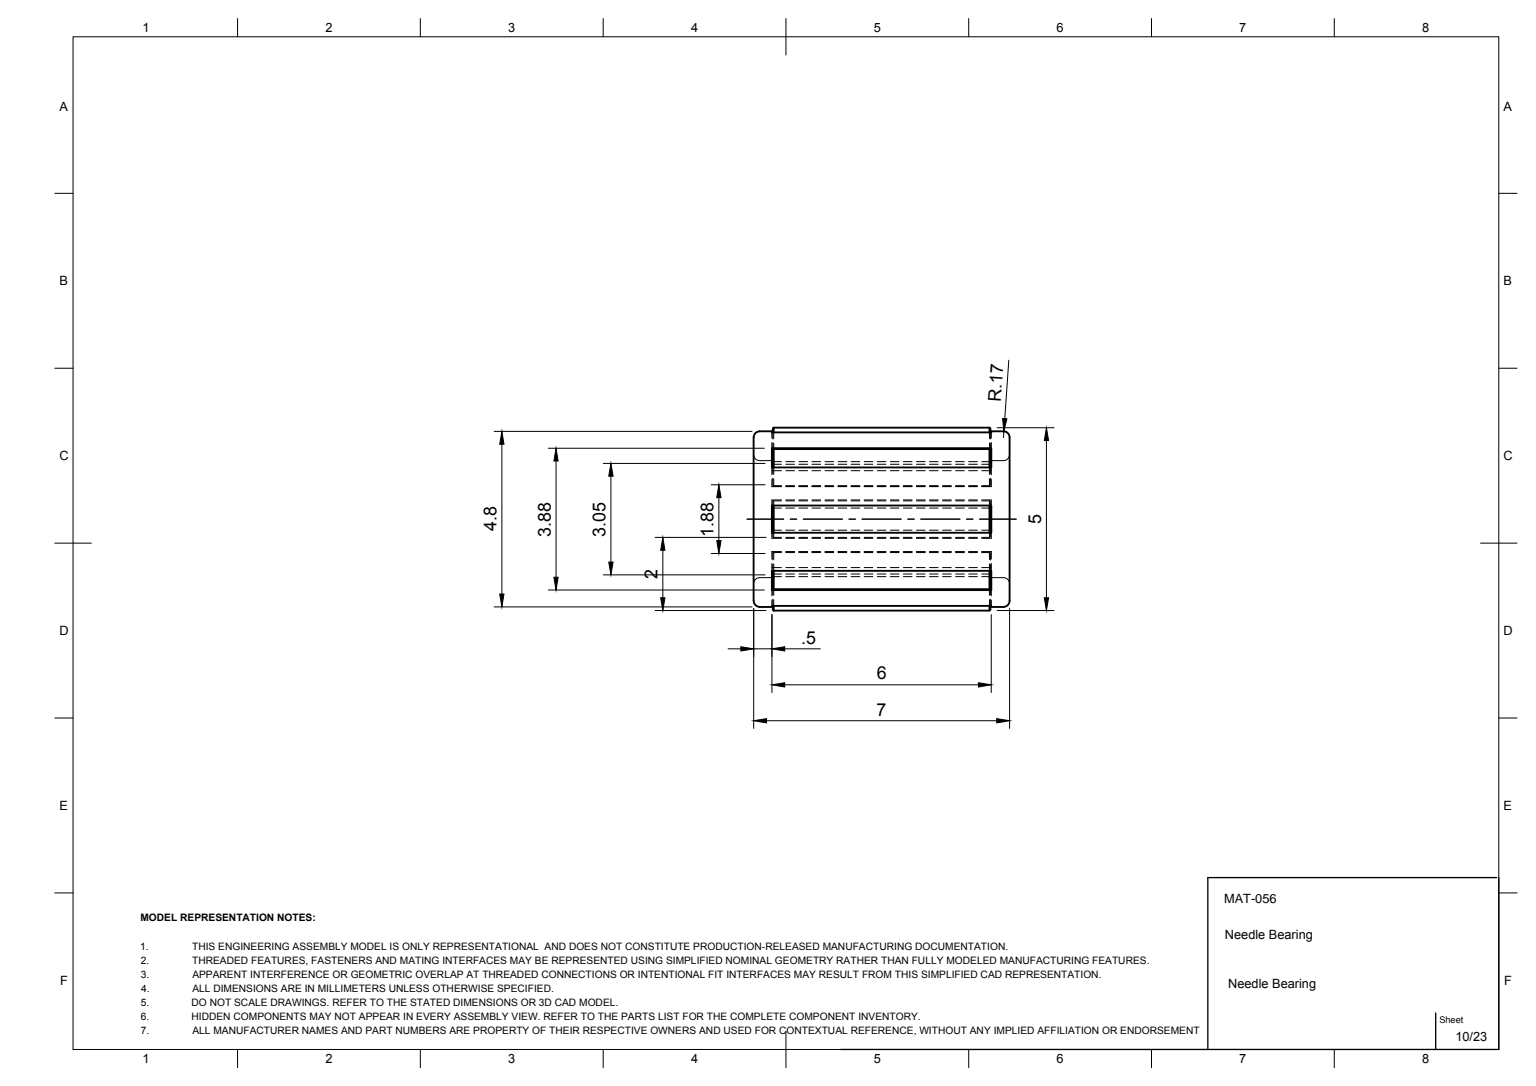
ISO-10303-21;
HEADER;
/* Generated by software containing ST-Developer
 * from STEP Tools, Inc. (www.steptools.com) 
 */

FILE_DESCRIPTION(
/* description */ (''),
/* implementation_level */ '2;1');

FILE_NAME(
/* name */ 'Needle Bearing.step',
/* time_stamp */ '2026-10-28T16:47:13+01:00',
/* author */ (''),
/* organization */ (''),
/* preprocessor_version */ 'ST-DEVELOPER v20.2',
/* originating_system */ 'Autodesk Translation Framework v15.17.0.0',
/* authorisation */ '');

FILE_SCHEMA (('AUTOMOTIVE_DESIGN { 1 0 10303 214 3 1 1 }'));
ENDSEC;

DATA;
#10=MECHANICAL_DESIGN_GEOMETRIC_PRESENTATION_REPRESENTATION('',(#4578,#4579,#4580,#4581,#4582,#4583,#4584,#4585,#4586),#459242);
#1858=TOROIDAL_SURFACE('',#98857,1.76666666666667,0.166666666666667);
#1859=TOROIDAL_SURFACE('',#98884,2.23333333333333,0.166666666666667);
#1860=TOROIDAL_SURFACE('',#98908,2.23333333333333,0.166666666666667);
#1861=TOROIDAL_SURFACE('',#98913,1.76666666666667,0.166666666666667);
#4413=SHAPE_REPRESENTATION_RELATIONSHIP('SRR','None',#459338,#4434);
#4434=ADVANCED_BREP_SHAPE_REPRESENTATION('',(#4458,#4459,#4460,#4461,#4462,
#4463,#4464,#4465,#4466),#459227);
#4458=MANIFOLD_SOLID_BREP('Bearing body',#94636);
#4459=MANIFOLD_SOLID_BREP('Roller 1',#94637);
#4460=MANIFOLD_SOLID_BREP('Roller 2',#94638);
#4461=MANIFOLD_SOLID_BREP('Roller 3',#94639);
#4462=MANIFOLD_SOLID_BREP('Roller 4',#94640);
#4463=MANIFOLD_SOLID_BREP('Roller 5',#94641);
#4464=MANIFOLD_SOLID_BREP('Roller 6',#94642);
#4465=MANIFOLD_SOLID_BREP('Roller 7',#94643);
#4466=MANIFOLD_SOLID_BREP('Roller 8',#94644);
#4578=STYLED_ITEM('',(#459526),#4458);
#4579=STYLED_ITEM('',(#459526),#4459);
#4580=STYLED_ITEM('',(#459526),#4460);
#4581=STYLED_ITEM('',(#459526),#4461);
#4582=STYLED_ITEM('',(#459526),#4462);
#4583=STYLED_ITEM('',(#459526),#4463);
#4584=STYLED_ITEM('',(#459526),#4464);
#4585=STYLED_ITEM('',(#459526),#4465);
#4586=STYLED_ITEM('',(#459526),#4466);
#4861=CONICAL_SURFACE('',#98979,0.4875,0.785398163397448);
#4862=CONICAL_SURFACE('',#98985,0.4875,0.785398163397448);
#4863=CONICAL_SURFACE('',#98988,0.4875,0.785398163397492);
#4864=CONICAL_SURFACE('',#98994,0.4875,0.785398163397492);
#4865=CONICAL_SURFACE('',#98997,0.4875,0.785398163397448);
#4866=CONICAL_SURFACE('',#99003,0.4875,0.785398163397448);
#4867=CONICAL_SURFACE('',#99006,0.4875,0.78539816339745);
#4868=CONICAL_SURFACE('',#99012,0.4875,0.78539816339745);
#4869=CONICAL_SURFACE('',#99015,0.4875,0.785398163397448);
#4870=CONICAL_SURFACE('',#99021,0.4875,0.785398163397448);
#4871=CONICAL_SURFACE('',#99024,0.4875,0.78539816339745);
#4872=CONICAL_SURFACE('',#99030,0.4875,0.78539816339745);
#4873=CONICAL_SURFACE('',#99033,0.4875,0.785398163397448);
#4874=CONICAL_SURFACE('',#99039,0.4875,0.785398163397448);
#4875=CONICAL_SURFACE('',#99042,0.4875,0.78539816339745);
#4876=CONICAL_SURFACE('',#99048,0.4875,0.78539816339745);
#5193=FACE_BOUND('',#14123,.T.);
#5194=FACE_BOUND('',#14125,.T.);
#5195=FACE_BOUND('',#14126,.T.);
#5196=FACE_BOUND('',#14127,.T.);
#5197=FACE_BOUND('',#14128,.T.);
#5198=FACE_BOUND('',#14129,.T.);
#5199=FACE_BOUND('',#14130,.T.);
#5200=FACE_BOUND('',#14131,.T.);
#5201=FACE_BOUND('',#14134,.T.);
#5202=FACE_BOUND('',#14135,.T.);
#5203=FACE_BOUND('',#14136,.T.);
#5204=FACE_BOUND('',#14137,.T.);
#5205=FACE_BOUND('',#14138,.T.);
#5206=FACE_BOUND('',#14139,.T.);
#5207=FACE_BOUND('',#14140,.T.);
#5208=FACE_BOUND('',#14143,.T.);
#5650=PLANE('',#98861);
#5651=PLANE('',#98911);
#5652=PLANE('',#98915);
#5653=PLANE('',#98920);
#5654=PLANE('',#98923);
#5655=PLANE('',#98928);
#5656=PLANE('',#98931);
#5657=PLANE('',#98936);
#5658=PLANE('',#98939);
#5659=PLANE('',#98944);
#5660=PLANE('',#98947);
#5661=PLANE('',#98952);
#5662=PLANE('',#98955);
#5663=PLANE('',#98960);
#5664=PLANE('',#98963);
#5665=PLANE('',#98968);
#5666=PLANE('',#98971);
#5667=PLANE('',#98976);
#5668=PLANE('',#98984);
#5669=PLANE('',#98987);
#5670=PLANE('',#98993);
#5671=PLANE('',#98996);
#5672=PLANE('',#99002);
#5673=PLANE('',#99005);
#5674=PLANE('',#99011);
#5675=PLANE('',#99014);
#5676=PLANE('',#99020);
#5677=PLANE('',#99023);
#5678=PLANE('',#99029);
#5679=PLANE('',#99032);
#5680=PLANE('',#99038);
#5681=PLANE('',#99041);
#5682=PLANE('',#99047);
#5683=PLANE('',#99050);
#8233=FACE_OUTER_BOUND('',#14121,.T.);
#8234=FACE_OUTER_BOUND('',#14122,.T.);
#8235=FACE_OUTER_BOUND('',#14124,.T.);
#8236=FACE_OUTER_BOUND('',#14132,.T.);
#8237=FACE_OUTER_BOUND('',#14133,.T.);
#8238=FACE_OUTER_BOUND('',#14141,.T.);
#8239=FACE_OUTER_BOUND('',#14142,.T.);
#8240=FACE_OUTER_BOUND('',#14144,.T.);
#8241=FACE_OUTER_BOUND('',#14145,.T.);
#8242=FACE_OUTER_BOUND('',#14146,.T.);
#8243=FACE_OUTER_BOUND('',#14147,.T.);
#8244=FACE_OUTER_BOUND('',#14148,.T.);
#8245=FACE_OUTER_BOUND('',#14149,.T.);
#8246=FACE_OUTER_BOUND('',#14150,.T.);
#8247=FACE_OUTER_BOUND('',#14151,.T.);
#8248=FACE_OUTER_BOUND('',#14152,.T.);
#8249=FACE_OUTER_BOUND('',#14153,.T.);
#8250=FACE_OUTER_BOUND('',#14154,.T.);
#8251=FACE_OUTER_BOUND('',#14155,.T.);
#8252=FACE_OUTER_BOUND('',#14156,.T.);
#8253=FACE_OUTER_BOUND('',#14157,.T.);
#8254=FACE_OUTER_BOUND('',#14158,.T.);
#8255=FACE_OUTER_BOUND('',#14159,.T.);
#8256=FACE_OUTER_BOUND('',#14160,.T.);
#8257=FACE_OUTER_BOUND('',#14161,.T.);
#8258=FACE_OUTER_BOUND('',#14162,.T.);
#8259=FACE_OUTER_BOUND('',#14163,.T.);
#8260=FACE_OUTER_BOUND('',#14164,.T.);
#8261=FACE_OUTER_BOUND('',#14165,.T.);
#8262=FACE_OUTER_BOUND('',#14166,.T.);
#8263=FACE_OUTER_BOUND('',#14167,.T.);
#8264=FACE_OUTER_BOUND('',#14168,.T.);
#8265=FACE_OUTER_BOUND('',#14169,.T.);
#8266=FACE_OUTER_BOUND('',#14170,.T.);
#8267=FACE_OUTER_BOUND('',#14171,.T.);
#8268=FACE_OUTER_BOUND('',#14172,.T.);
#8269=FACE_OUTER_BOUND('',#14173,.T.);
#8270=FACE_OUTER_BOUND('',#14174,.T.);
#8271=FACE_OUTER_BOUND('',#14175,.T.);
#8272=FACE_OUTER_BOUND('',#14176,.T.);
#8273=FACE_OUTER_BOUND('',#14177,.T.);
#8274=FACE_OUTER_BOUND('',#14178,.T.);
#8275=FACE_OUTER_BOUND('',#14179,.T.);
#8276=FACE_OUTER_BOUND('',#14180,.T.);
#8277=FACE_OUTER_BOUND('',#14181,.T.);
#8278=FACE_OUTER_BOUND('',#14182,.T.);
#8279=FACE_OUTER_BOUND('',#14183,.T.);
#8280=FACE_OUTER_BOUND('',#14184,.T.);
#8281=FACE_OUTER_BOUND('',#14185,.T.);
#8282=FACE_OUTER_BOUND('',#14186,.T.);
#8283=FACE_OUTER_BOUND('',#14187,.T.);
#8284=FACE_OUTER_BOUND('',#14188,.T.);
#8285=FACE_OUTER_BOUND('',#14189,.T.);
#8286=FACE_OUTER_BOUND('',#14190,.T.);
#8287=FACE_OUTER_BOUND('',#14191,.T.);
#8288=FACE_OUTER_BOUND('',#14192,.T.);
#8289=FACE_OUTER_BOUND('',#14193,.T.);
#8290=FACE_OUTER_BOUND('',#14194,.T.);
#8291=FACE_OUTER_BOUND('',#14195,.T.);
#8292=FACE_OUTER_BOUND('',#14196,.T.);
#8293=FACE_OUTER_BOUND('',#14197,.T.);
#8294=FACE_OUTER_BOUND('',#14198,.T.);
#8295=FACE_OUTER_BOUND('',#14199,.T.);
#8296=FACE_OUTER_BOUND('',#14200,.T.);
#8297=FACE_OUTER_BOUND('',#14201,.T.);
#8298=FACE_OUTER_BOUND('',#14202,.T.);
#8299=FACE_OUTER_BOUND('',#14203,.T.);
#8300=FACE_OUTER_BOUND('',#14204,.T.);
#8301=FACE_OUTER_BOUND('',#14205,.T.);
#8302=FACE_OUTER_BOUND('',#14206,.T.);
#8303=FACE_OUTER_BOUND('',#14207,.T.);
#8304=FACE_OUTER_BOUND('',#14208,.T.);
#8305=FACE_OUTER_BOUND('',#14209,.T.);
#8306=FACE_OUTER_BOUND('',#14210,.T.);
#8307=FACE_OUTER_BOUND('',#14211,.T.);
#8308=FACE_OUTER_BOUND('',#14212,.T.);
#8309=FACE_OUTER_BOUND('',#14213,.T.);
#8310=FACE_OUTER_BOUND('',#14214,.T.);
#8311=FACE_OUTER_BOUND('',#14215,.T.);
#8312=FACE_OUTER_BOUND('',#14216,.T.);
#14121=EDGE_LOOP('',(#68422,#68423,#68424,#68425));
#14122=EDGE_LOOP('',(#68426));
#14123=EDGE_LOOP('',(#68427));
#14124=EDGE_LOOP('',(#68428,#68429,#68430,#68431,#68432,#68433,#68434,#68435,
#68436,#68437,#68438,#68439,#68440));
#14125=EDGE_LOOP('',(#68441,#68442,#68443,#68444));
#14126=EDGE_LOOP('',(#68445,#68446,#68447,#68448));
#14127=EDGE_LOOP('',(#68449,#68450,#68451,#68452));
#14128=EDGE_LOOP('',(#68453,#68454,#68455,#68456));
#14129=EDGE_LOOP('',(#68457,#68458,#68459,#68460));
#14130=EDGE_LOOP('',(#68461,#68462,#68463,#68464));
#14131=EDGE_LOOP('',(#68465,#68466,#68467,#68468));
#14132=EDGE_LOOP('',(#68469,#68470,#68471,#68472,#68473));
#14133=EDGE_LOOP('',(#68474,#68475,#68476,#68477,#68478,#68479,#68480,#68481,
#68482,#68483,#68484,#68485,#68486));
#14134=EDGE_LOOP('',(#68487,#68488,#68489,#68490));
#14135=EDGE_LOOP('',(#68491,#68492,#68493,#68494));
#14136=EDGE_LOOP('',(#68495,#68496,#68497,#68498));
#14137=EDGE_LOOP('',(#68499,#68500,#68501,#68502));
#14138=EDGE_LOOP('',(#68503,#68504,#68505,#68506));
#14139=EDGE_LOOP('',(#68507,#68508,#68509,#68510));
#14140=EDGE_LOOP('',(#68511,#68512,#68513,#68514));
#14141=EDGE_LOOP('',(#68515,#68516,#68517,#68518));
#14142=EDGE_LOOP('',(#68519));
#14143=EDGE_LOOP('',(#68520));
#14144=EDGE_LOOP('',(#68521,#68522,#68523,#68524,#68525));
#14145=EDGE_LOOP('',(#68526,#68527,#68528,#68529));
#14146=EDGE_LOOP('',(#68530,#68531,#68532,#68533));
#14147=EDGE_LOOP('',(#68534,#68535,#68536,#68537));
#14148=EDGE_LOOP('',(#68538,#68539,#68540,#68541));
#14149=EDGE_LOOP('',(#68542,#68543,#68544,#68545));
#14150=EDGE_LOOP('',(#68546,#68547,#68548,#68549));
#14151=EDGE_LOOP('',(#68550,#68551,#68552,#68553));
#14152=EDGE_LOOP('',(#68554,#68555,#68556,#68557));
#14153=EDGE_LOOP('',(#68558,#68559,#68560,#68561));
#14154=EDGE_LOOP('',(#68562,#68563,#68564,#68565));
#14155=EDGE_LOOP('',(#68566,#68567,#68568,#68569));
#14156=EDGE_LOOP('',(#68570,#68571,#68572,#68573));
#14157=EDGE_LOOP('',(#68574,#68575,#68576,#68577,#68578,#68579));
#14158=EDGE_LOOP('',(#68580,#68581,#68582,#68583));
#14159=EDGE_LOOP('',(#68584,#68585,#68586,#68587,#68588,#68589));
#14160=EDGE_LOOP('',(#68590,#68591,#68592,#68593));
#14161=EDGE_LOOP('',(#68594,#68595,#68596,#68597));
#14162=EDGE_LOOP('',(#68598,#68599,#68600,#68601));
#14163=EDGE_LOOP('',(#68602,#68603,#68604,#68605));
#14164=EDGE_LOOP('',(#68606,#68607,#68608,#68609));
#14165=EDGE_LOOP('',(#68610,#68611,#68612,#68613));
#14166=EDGE_LOOP('',(#68614,#68615,#68616,#68617));
#14167=EDGE_LOOP('',(#68618,#68619,#68620,#68621));
#14168=EDGE_LOOP('',(#68622,#68623,#68624,#68625));
#14169=EDGE_LOOP('',(#68626,#68627,#68628,#68629));
#14170=EDGE_LOOP('',(#68630,#68631,#68632,#68633));
#14171=EDGE_LOOP('',(#68634,#68635,#68636,#68637));
#14172=EDGE_LOOP('',(#68638,#68639,#68640,#68641));
#14173=EDGE_LOOP('',(#68642,#68643,#68644,#68645));
#14174=EDGE_LOOP('',(#68646,#68647,#68648,#68649));
#14175=EDGE_LOOP('',(#68650,#68651,#68652,#68653));
#14176=EDGE_LOOP('',(#68654,#68655,#68656,#68657));
#14177=EDGE_LOOP('',(#68658,#68659,#68660,#68661));
#14178=EDGE_LOOP('',(#68662,#68663,#68664,#68665));
#14179=EDGE_LOOP('',(#68666));
#14180=EDGE_LOOP('',(#68667,#68668,#68669,#68670));
#14181=EDGE_LOOP('',(#68671));
#14182=EDGE_LOOP('',(#68672,#68673,#68674,#68675));
#14183=EDGE_LOOP('',(#68676,#68677,#68678,#68679));
#14184=EDGE_LOOP('',(#68680));
#14185=EDGE_LOOP('',(#68681,#68682,#68683,#68684));
#14186=EDGE_LOOP('',(#68685));
#14187=EDGE_LOOP('',(#68686,#68687,#68688,#68689));
#14188=EDGE_LOOP('',(#68690,#68691,#68692,#68693));
#14189=EDGE_LOOP('',(#68694));
#14190=EDGE_LOOP('',(#68695,#68696,#68697,#68698));
#14191=EDGE_LOOP('',(#68699));
#14192=EDGE_LOOP('',(#68700,#68701,#68702,#68703));
#14193=EDGE_LOOP('',(#68704,#68705,#68706,#68707));
#14194=EDGE_LOOP('',(#68708));
#14195=EDGE_LOOP('',(#68709,#68710,#68711,#68712));
#14196=EDGE_LOOP('',(#68713));
#14197=EDGE_LOOP('',(#68714,#68715,#68716,#68717));
#14198=EDGE_LOOP('',(#68718,#68719,#68720,#68721));
#14199=EDGE_LOOP('',(#68722));
#14200=EDGE_LOOP('',(#68723,#68724,#68725,#68726));
#14201=EDGE_LOOP('',(#68727));
#14202=EDGE_LOOP('',(#68728,#68729,#68730,#68731));
#14203=EDGE_LOOP('',(#68732,#68733,#68734,#68735));
#14204=EDGE_LOOP('',(#68736));
#14205=EDGE_LOOP('',(#68737,#68738,#68739,#68740));
#14206=EDGE_LOOP('',(#68741));
#14207=EDGE_LOOP('',(#68742,#68743,#68744,#68745));
#14208=EDGE_LOOP('',(#68746,#68747,#68748,#68749));
#14209=EDGE_LOOP('',(#68750));
#14210=EDGE_LOOP('',(#68751,#68752,#68753,#68754));
#14211=EDGE_LOOP('',(#68755));
#14212=EDGE_LOOP('',(#68756,#68757,#68758,#68759));
#14213=EDGE_LOOP('',(#68760,#68761,#68762,#68763));
#14214=EDGE_LOOP('',(#68764));
#14215=EDGE_LOOP('',(#68765,#68766,#68767,#68768));
#14216=EDGE_LOOP('',(#68769));
#20404=CIRCLE('',#98858,1.76666666666667);
#20405=CIRCLE('',#98859,0.166666666666667);
#20406=CIRCLE('',#98860,1.6);
#20407=CIRCLE('',#98862,2.23333333333333);
#20408=CIRCLE('',#98864,1.6);
#20409=CIRCLE('',#98865,1.6);
#20410=CIRCLE('',#98866,1.6);
#20411=CIRCLE('',#98867,1.6);
#20412=CIRCLE('',#98868,1.6);
#20413=CIRCLE('',#98869,1.6);
#20414=CIRCLE('',#98870,1.6);
#20415=CIRCLE('',#98871,1.6);
#20416=CIRCLE('',#98872,1.6);
#20417=CIRCLE('',#98873,1.6);
#20418=CIRCLE('',#98874,1.6);
#20419=CIRCLE('',#98875,1.6);
#20420=CIRCLE('',#98876,1.6);
#20421=CIRCLE('',#98877,1.6);
#20422=CIRCLE('',#98878,1.6);
#20423=CIRCLE('',#98879,1.6);
#20424=CIRCLE('',#98880,1.6);
#20425=CIRCLE('',#98881,1.6);
#20426=CIRCLE('',#98882,1.6);
#20427=CIRCLE('',#98883,1.6);
#20428=CIRCLE('',#98885,0.166666666666667);
#20429=CIRCLE('',#98886,2.4);
#20430=CIRCLE('',#98887,2.4);
#20431=CIRCLE('',#98889,2.4);
#20432=CIRCLE('',#98890,2.4);
#20433=CIRCLE('',#98891,2.4);
#20434=CIRCLE('',#98892,2.4);
#20435=CIRCLE('',#98893,2.4);
#20436=CIRCLE('',#98894,2.4);
#20437=CIRCLE('',#98895,2.4);
#20438=CIRCLE('',#98896,2.4);
#20439=CIRCLE('',#98897,2.4);
#20440=CIRCLE('',#98898,2.4);
#20441=CIRCLE('',#98899,2.4);
#20442=CIRCLE('',#98900,2.4);
#20443=CIRCLE('',#98901,2.4);
#20444=CIRCLE('',#98902,2.4);
#20445=CIRCLE('',#98903,2.4);
#20446=CIRCLE('',#98904,2.4);
#20447=CIRCLE('',#98905,2.4);
#20448=CIRCLE('',#98906,2.4);
#20449=CIRCLE('',#98907,2.4);
#20450=CIRCLE('',#98909,2.23333333333333);
#20451=CIRCLE('',#98910,0.166666666666667);
#20452=CIRCLE('',#98912,1.76666666666667);
#20453=CIRCLE('',#98914,0.166666666666667);
#20454=CIRCLE('',#98916,0.525);
#20455=CIRCLE('',#98917,0.525);
#20456=CIRCLE('',#98919,0.525);
#20457=CIRCLE('',#98921,0.525);
#20458=CIRCLE('',#98924,0.525);
#20459=CIRCLE('',#98925,0.525);
#20460=CIRCLE('',#98927,0.525);
#20461=CIRCLE('',#98929,0.525);
#20462=CIRCLE('',#98932,0.525);
#20463=CIRCLE('',#98933,0.525);
#20464=CIRCLE('',#98935,0.525);
#20465=CIRCLE('',#98937,0.525);
#20466=CIRCLE('',#98940,0.525);
#20467=CIRCLE('',#98941,0.525);
#20468=CIRCLE('',#98943,0.525);
#20469=CIRCLE('',#98945,0.525);
#20470=CIRCLE('',#98948,0.525);
#20471=CIRCLE('',#98949,0.525);
#20472=CIRCLE('',#98951,0.525);
#20473=CIRCLE('',#98953,0.525);
#20474=CIRCLE('',#98956,0.525);
#20475=CIRCLE('',#98957,0.525);
#20476=CIRCLE('',#98959,0.525);
#20477=CIRCLE('',#98961,0.525);
#20478=CIRCLE('',#98964,0.525);
#20479=CIRCLE('',#98965,0.525);
#20480=CIRCLE('',#98967,0.525);
#20481=CIRCLE('',#98969,0.525);
#20482=CIRCLE('',#98972,0.525);
#20483=CIRCLE('',#98973,0.525);
#20484=CIRCLE('',#98975,0.525);
#20485=CIRCLE('',#98977,0.525);
#20486=CIRCLE('',#98980,0.5);
#20487=CIRCLE('',#98981,0.475);
#20488=CIRCLE('',#98983,0.5);
#20489=CIRCLE('',#98986,0.475);
#20490=CIRCLE('',#98989,0.5);
#20491=CIRCLE('',#98990,0.475);
#20492=CIRCLE('',#98992,0.5);
#20493=CIRCLE('',#98995,0.475);
#20494=CIRCLE('',#98998,0.5);
#20495=CIRCLE('',#98999,0.475);
#20496=CIRCLE('',#99001,0.5);
#20497=CIRCLE('',#99004,0.475);
#20498=CIRCLE('',#99007,0.5);
#20499=CIRCLE('',#99008,0.475);
#20500=CIRCLE('',#99010,0.5);
#20501=CIRCLE('',#99013,0.475);
#20502=CIRCLE('',#99016,0.5);
#20503=CIRCLE('',#99017,0.475);
#20504=CIRCLE('',#99019,0.5);
#20505=CIRCLE('',#99022,0.475);
#20506=CIRCLE('',#99025,0.5);
#20507=CIRCLE('',#99026,0.475);
#20508=CIRCLE('',#99028,0.5);
#20509=CIRCLE('',#99031,0.475);
#20510=CIRCLE('',#99034,0.5);
#20511=CIRCLE('',#99035,0.475);
#20512=CIRCLE('',#99037,0.5);
#20513=CIRCLE('',#99040,0.475);
#20514=CIRCLE('',#99043,0.5);
#20515=CIRCLE('',#99044,0.475);
#20516=CIRCLE('',#99046,0.5);
#20517=CIRCLE('',#99049,0.475);
#28838=LINE('',#358172,#32640);
#28839=LINE('',#358176,#32641);
#28840=LINE('',#358180,#32642);
#28841=LINE('',#358187,#32643);
#28842=LINE('',#358193,#32644);
#28843=LINE('',#358196,#32645);
#28844=LINE('',#358201,#32646);
#28845=LINE('',#358204,#32647);
#28846=LINE('',#358209,#32648);
#28847=LINE('',#358212,#32649);
#28848=LINE('',#358217,#32650);
#28849=LINE('',#358220,#32651);
#28850=LINE('',#358225,#32652);
#28851=LINE('',#358228,#32653);
#28852=LINE('',#358233,#32654);
#28853=LINE('',#358236,#32655);
#28854=LINE('',#358241,#32656);
#28855=LINE('',#358244,#32657);
#28856=LINE('',#358255,#32658);
#28857=LINE('',#358259,#32659);
#28858=LINE('',#358262,#32660);
#28859=LINE('',#358266,#32661);
#28860=LINE('',#358272,#32662);
#28861=LINE('',#358275,#32663);
#28862=LINE('',#358280,#32664);
#28863=LINE('',#358283,#32665);
#28864=LINE('',#358288,#32666);
#28865=LINE('',#358291,#32667);
#28866=LINE('',#358296,#32668);
#28867=LINE('',#358299,#32669);
#28868=LINE('',#358304,#32670);
#28869=LINE('',#358307,#32671);
#28870=LINE('',#358312,#32672);
#28871=LINE('',#358315,#32673);
#28872=LINE('',#358320,#32674);
#28873=LINE('',#358323,#32675);
#28874=LINE('',#358401,#32676);
#28875=LINE('',#358406,#32677);
#28876=LINE('',#358410,#32678);
#28877=LINE('',#358417,#32679);
#28878=LINE('',#358422,#32680);
#28879=LINE('',#358426,#32681);
#28880=LINE('',#358433,#32682);
#28881=LINE('',#358438,#32683);
#28882=LINE('',#358442,#32684);
#28883=LINE('',#358449,#32685);
#28884=LINE('',#358454,#32686);
#28885=LINE('',#358458,#32687);
#28886=LINE('',#358465,#32688);
#28887=LINE('',#358470,#32689);
#28888=LINE('',#358474,#32690);
#28889=LINE('',#358481,#32691);
#28890=LINE('',#358486,#32692);
#28891=LINE('',#358490,#32693);
#28892=LINE('',#358497,#32694);
#28893=LINE('',#358502,#32695);
#28894=LINE('',#358506,#32696);
#28895=LINE('',#358513,#32697);
#28896=LINE('',#358518,#32698);
#28897=LINE('',#358522,#32699);
#32640=VECTOR('',#115286,1.6);
#32641=VECTOR('',#115289,10.);
#32642=VECTOR('',#115292,1.6);
#32643=VECTOR('',#115299,10.);
#32644=VECTOR('',#115304,10.);
#32645=VECTOR('',#115307,10.);
#32646=VECTOR('',#115310,10.);
#32647=VECTOR('',#115313,10.);
#32648=VECTOR('',#115316,10.);
#32649=VECTOR('',#115319,10.);
#32650=VECTOR('',#115322,10.);
#32651=VECTOR('',#115325,10.);
#32652=VECTOR('',#115328,10.);
#32653=VECTOR('',#115331,10.);
#32654=VECTOR('',#115334,10.);
#32655=VECTOR('',#115337,10.);
#32656=VECTOR('',#115340,10.);
#32657=VECTOR('',#115343,10.);
#32658=VECTOR('',#115356,2.4);
#32659=VECTOR('',#115359,10.);
#32660=VECTOR('',#115362,2.4);
#32661=VECTOR('',#115365,10.);
#32662=VECTOR('',#115370,10.);
#32663=VECTOR('',#115373,10.);
#32664=VECTOR('',#115376,10.);
#32665=VECTOR('',#115379,10.);
#32666=VECTOR('',#115382,10.);
#32667=VECTOR('',#115385,10.);
#32668=VECTOR('',#115388,10.);
#32669=VECTOR('',#115391,10.);
#32670=VECTOR('',#115394,10.);
#32671=VECTOR('',#115397,10.);
#32672=VECTOR('',#115400,10.);
#32673=VECTOR('',#115403,10.);
#32674=VECTOR('',#115406,10.);
#32675=VECTOR('',#115409,10.);
#32676=VECTOR('',#115556,0.4875);
#32677=VECTOR('',#115563,0.5);
#32678=VECTOR('',#115568,0.4875);
#32679=VECTOR('',#115577,0.4875);
#32680=VECTOR('',#115584,0.5);
#32681=VECTOR('',#115589,0.4875);
#32682=VECTOR('',#115598,0.4875);
#32683=VECTOR('',#115605,0.5);
#32684=VECTOR('',#115610,0.4875);
#32685=VECTOR('',#115619,0.4875);
#32686=VECTOR('',#115626,0.5);
#32687=VECTOR('',#115631,0.4875);
#32688=VECTOR('',#115640,0.4875);
#32689=VECTOR('',#115647,0.5);
#32690=VECTOR('',#115652,0.4875);
#32691=VECTOR('',#115661,0.4875);
#32692=VECTOR('',#115668,0.5);
#32693=VECTOR('',#115673,0.4875);
#32694=VECTOR('',#115682,0.4875);
#32695=VECTOR('',#115689,0.5);
#32696=VECTOR('',#115694,0.4875);
#32697=VECTOR('',#115703,0.4875);
#32698=VECTOR('',#115710,0.5);
#32699=VECTOR('',#115715,0.4875);
#38018=VERTEX_POINT('',#358162);
#38019=VERTEX_POINT('',#358164);
#38020=VERTEX_POINT('',#358168);
#38021=VERTEX_POINT('',#358171);
#38022=VERTEX_POINT('',#358173);
#38023=VERTEX_POINT('',#358175);
#38024=VERTEX_POINT('',#358177);
#38025=VERTEX_POINT('',#358179);
#38026=VERTEX_POINT('',#358181);
#38027=VERTEX_POINT('',#358184);
#38028=VERTEX_POINT('',#358186);
#38029=VERTEX_POINT('',#358189);
#38030=VERTEX_POINT('',#358190);
#38031=VERTEX_POINT('',#358192);
#38032=VERTEX_POINT('',#358194);
#38033=VERTEX_POINT('',#358197);
#38034=VERTEX_POINT('',#358198);
#38035=VERTEX_POINT('',#358200);
#38036=VERTEX_POINT('',#358202);
#38037=VERTEX_POINT('',#358205);
#38038=VERTEX_POINT('',#358206);
#38039=VERTEX_POINT('',#358208);
#38040=VERTEX_POINT('',#358210);
#38041=VERTEX_POINT('',#358213);
#38042=VERTEX_POINT('',#358214);
#38043=VERTEX_POINT('',#358216);
#38044=VERTEX_POINT('',#358218);
#38045=VERTEX_POINT('',#358221);
#38046=VERTEX_POINT('',#358222);
#38047=VERTEX_POINT('',#358224);
#38048=VERTEX_POINT('',#358226);
#38049=VERTEX_POINT('',#358229);
#38050=VERTEX_POINT('',#358230);
#38051=VERTEX_POINT('',#358232);
#38052=VERTEX_POINT('',#358234);
#38053=VERTEX_POINT('',#358237);
#38054=VERTEX_POINT('',#358238);
#38055=VERTEX_POINT('',#358240);
#38056=VERTEX_POINT('',#358242);
#38057=VERTEX_POINT('',#358246);
#38058=VERTEX_POINT('',#358248);
#38059=VERTEX_POINT('',#358252);
#38060=VERTEX_POINT('',#358254);
#38061=VERTEX_POINT('',#358256);
#38062=VERTEX_POINT('',#358258);
#38063=VERTEX_POINT('',#358260);
#38064=VERTEX_POINT('',#358263);
#38065=VERTEX_POINT('',#358265);
#38066=VERTEX_POINT('',#358268);
#38067=VERTEX_POINT('',#358269);
#38068=VERTEX_POINT('',#358271);
#38069=VERTEX_POINT('',#358273);
#38070=VERTEX_POINT('',#358276);
#38071=VERTEX_POINT('',#358277);
#38072=VERTEX_POINT('',#358279);
#38073=VERTEX_POINT('',#358281);
#38074=VERTEX_POINT('',#358284);
#38075=VERTEX_POINT('',#358285);
#38076=VERTEX_POINT('',#358287);
#38077=VERTEX_POINT('',#358289);
#38078=VERTEX_POINT('',#358292);
#38079=VERTEX_POINT('',#358293);
#38080=VERTEX_POINT('',#358295);
#38081=VERTEX_POINT('',#358297);
#38082=VERTEX_POINT('',#358300);
#38083=VERTEX_POINT('',#358301);
#38084=VERTEX_POINT('',#358303);
#38085=VERTEX_POINT('',#358305);
#38086=VERTEX_POINT('',#358308);
#38087=VERTEX_POINT('',#358309);
#38088=VERTEX_POINT('',#358311);
#38089=VERTEX_POINT('',#358313);
#38090=VERTEX_POINT('',#358316);
#38091=VERTEX_POINT('',#358317);
#38092=VERTEX_POINT('',#358319);
#38093=VERTEX_POINT('',#358321);
#38094=VERTEX_POINT('',#358325);
#38095=VERTEX_POINT('',#358329);
#38096=VERTEX_POINT('',#358398);
#38097=VERTEX_POINT('',#358400);
#38098=VERTEX_POINT('',#358404);
#38099=VERTEX_POINT('',#358409);
#38100=VERTEX_POINT('',#358414);
#38101=VERTEX_POINT('',#358416);
#38102=VERTEX_POINT('',#358420);
#38103=VERTEX_POINT('',#358425);
#38104=VERTEX_POINT('',#358430);
#38105=VERTEX_POINT('',#358432);
#38106=VERTEX_POINT('',#358436);
#38107=VERTEX_POINT('',#358441);
#38108=VERTEX_POINT('',#358446);
#38109=VERTEX_POINT('',#358448);
#38110=VERTEX_POINT('',#358452);
#38111=VERTEX_POINT('',#358457);
#38112=VERTEX_POINT('',#358462);
#38113=VERTEX_POINT('',#358464);
#38114=VERTEX_POINT('',#358468);
#38115=VERTEX_POINT('',#358473);
#38116=VERTEX_POINT('',#358478);
#38117=VERTEX_POINT('',#358480);
#38118=VERTEX_POINT('',#358484);
#38119=VERTEX_POINT('',#358489);
#38120=VERTEX_POINT('',#358494);
#38121=VERTEX_POINT('',#358496);
#38122=VERTEX_POINT('',#358500);
#38123=VERTEX_POINT('',#358505);
#38124=VERTEX_POINT('',#358510);
#38125=VERTEX_POINT('',#358512);
#38126=VERTEX_POINT('',#358516);
#38127=VERTEX_POINT('',#358521);
#48713=EDGE_CURVE('',#38018,#38018,#20404,.T.);
#48714=EDGE_CURVE('',#38018,#38019,#20405,.T.);
#48715=EDGE_CURVE('',#38019,#38019,#20406,.T.);
#48716=EDGE_CURVE('',#38020,#38020,#20407,.T.);
#48717=EDGE_CURVE('',#38019,#38021,#28838,.T.);
#48718=EDGE_CURVE('',#38021,#38022,#20408,.T.);
#48719=EDGE_CURVE('',#38022,#38023,#28839,.T.);
#48720=EDGE_CURVE('',#38023,#38024,#20409,.T.);
#48721=EDGE_CURVE('',#38024,#38025,#28840,.T.);
#48722=EDGE_CURVE('',#38026,#38025,#20410,.T.);
#48723=EDGE_CURVE('',#38025,#38026,#20411,.T.);
#48724=EDGE_CURVE('',#38024,#38027,#20412,.T.);
#48725=EDGE_CURVE('',#38027,#38028,#28841,.T.);
#48726=EDGE_CURVE('',#38028,#38021,#20413,.T.);
#48727=EDGE_CURVE('',#38029,#38030,#20414,.T.);
#48728=EDGE_CURVE('',#38030,#38031,#28842,.T.);
#48729=EDGE_CURVE('',#38031,#38032,#20415,.T.);
#48730=EDGE_CURVE('',#38032,#38029,#28843,.T.);
#48731=EDGE_CURVE('',#38033,#38034,#20416,.T.);
#48732=EDGE_CURVE('',#38034,#38035,#28844,.T.);
#48733=EDGE_CURVE('',#38035,#38036,#20417,.T.);
#48734=EDGE_CURVE('',#38036,#38033,#28845,.T.);
#48735=EDGE_CURVE('',#38037,#38038,#20418,.T.);
#48736=EDGE_CURVE('',#38038,#38039,#28846,.T.);
#48737=EDGE_CURVE('',#38039,#38040,#20419,.T.);
#48738=EDGE_CURVE('',#38040,#38037,#28847,.T.);
#48739=EDGE_CURVE('',#38041,#38042,#20420,.T.);
#48740=EDGE_CURVE('',#38042,#38043,#28848,.T.);
#48741=EDGE_CURVE('',#38043,#38044,#20421,.T.);
#48742=EDGE_CURVE('',#38044,#38041,#28849,.T.);
#48743=EDGE_CURVE('',#38045,#38046,#20422,.T.);
#48744=EDGE_CURVE('',#38046,#38047,#28850,.T.);
#48745=EDGE_CURVE('',#38047,#38048,#20423,.T.);
#48746=EDGE_CURVE('',#38048,#38045,#28851,.T.);
#48747=EDGE_CURVE('',#38049,#38050,#20424,.T.);
#48748=EDGE_CURVE('',#38050,#38051,#28852,.T.);
#48749=EDGE_CURVE('',#38051,#38052,#20425,.T.);
#48750=EDGE_CURVE('',#38052,#38049,#28853,.T.);
#48751=EDGE_CURVE('',#38053,#38054,#20426,.T.);
#48752=EDGE_CURVE('',#38054,#38055,#28854,.T.);
#48753=EDGE_CURVE('',#38055,#38056,#20427,.T.);
#48754=EDGE_CURVE('',#38056,#38053,#28855,.T.);
#48755=EDGE_CURVE('',#38020,#38057,#20428,.T.);
#48756=EDGE_CURVE('',#38057,#38058,#20429,.T.);
#48757=EDGE_CURVE('',#38058,#38057,#20430,.T.);
#48758=EDGE_CURVE('',#38059,#38059,#20431,.T.);
#48759=EDGE_CURVE('',#38059,#38060,#28856,.T.);
#48760=EDGE_CURVE('',#38060,#38061,#20432,.T.);
#48761=EDGE_CURVE('',#38061,#38062,#28857,.T.);
#48762=EDGE_CURVE('',#38062,#38063,#20433,.T.);
#48763=EDGE_CURVE('',#38063,#38058,#28858,.T.);
#48764=EDGE_CURVE('',#38063,#38064,#20434,.T.);
#48765=EDGE_CURVE('',#38064,#38065,#28859,.T.);
#48766=EDGE_CURVE('',#38065,#38060,#20435,.T.);
#48767=EDGE_CURVE('',#38066,#38067,#20436,.T.);
#48768=EDGE_CURVE('',#38067,#38068,#28860,.T.);
#48769=EDGE_CURVE('',#38068,#38069,#20437,.T.);
#48770=EDGE_CURVE('',#38069,#38066,#28861,.T.);
#48771=EDGE_CURVE('',#38070,#38071,#20438,.T.);
#48772=EDGE_CURVE('',#38071,#38072,#28862,.T.);
#48773=EDGE_CURVE('',#38072,#38073,#20439,.T.);
#48774=EDGE_CURVE('',#38073,#38070,#28863,.T.);
#48775=EDGE_CURVE('',#38074,#38075,#20440,.T.);
#48776=EDGE_CURVE('',#38075,#38076,#28864,.T.);
#48777=EDGE_CURVE('',#38076,#38077,#20441,.T.);
#48778=EDGE_CURVE('',#38077,#38074,#28865,.T.);
#48779=EDGE_CURVE('',#38078,#38079,#20442,.T.);
#48780=EDGE_CURVE('',#38079,#38080,#28866,.T.);
#48781=EDGE_CURVE('',#38080,#38081,#20443,.T.);
#48782=EDGE_CURVE('',#38081,#38078,#28867,.T.);
#48783=EDGE_CURVE('',#38082,#38083,#20444,.T.);
#48784=EDGE_CURVE('',#38083,#38084,#28868,.T.);
#48785=EDGE_CURVE('',#38084,#38085,#20445,.T.);
#48786=EDGE_CURVE('',#38085,#38082,#28869,.T.);
#48787=EDGE_CURVE('',#38086,#38087,#20446,.T.);
#48788=EDGE_CURVE('',#38087,#38088,#28870,.T.);
#48789=EDGE_CURVE('',#38088,#38089,#20447,.T.);
#48790=EDGE_CURVE('',#38089,#38086,#28871,.T.);
#48791=EDGE_CURVE('',#38090,#38091,#20448,.T.);
#48792=EDGE_CURVE('',#38091,#38092,#28872,.T.);
#48793=EDGE_CURVE('',#38092,#38093,#20449,.T.);
#48794=EDGE_CURVE('',#38093,#38090,#28873,.T.);
#48795=EDGE_CURVE('',#38094,#38094,#20450,.T.);
#48796=EDGE_CURVE('',#38094,#38059,#20451,.T.);
#48797=EDGE_CURVE('',#38095,#38095,#20452,.T.);
#48798=EDGE_CURVE('',#38095,#38026,#20453,.T.);
#48799=EDGE_CURVE('',#38069,#38031,#20454,.T.);
#48800=EDGE_CURVE('',#38032,#38068,#20455,.T.);
#48801=EDGE_CURVE('',#38067,#38029,#20456,.T.);
#48802=EDGE_CURVE('',#38030,#38066,#20457,.T.);
#48803=EDGE_CURVE('',#38073,#38035,#20458,.T.);
#48804=EDGE_CURVE('',#38036,#38072,#20459,.T.);
#48805=EDGE_CURVE('',#38071,#38033,#20460,.T.);
#48806=EDGE_CURVE('',#38034,#38070,#20461,.T.);
#48807=EDGE_CURVE('',#38077,#38039,#20462,.T.);
#48808=EDGE_CURVE('',#38040,#38076,#20463,.T.);
#48809=EDGE_CURVE('',#38075,#38037,#20464,.T.);
#48810=EDGE_CURVE('',#38038,#38074,#20465,.T.);
#48811=EDGE_CURVE('',#38061,#38023,#20466,.T.);
#48812=EDGE_CURVE('',#38027,#38065,#20467,.T.);
#48813=EDGE_CURVE('',#38064,#38028,#20468,.T.);
#48814=EDGE_CURVE('',#38022,#38062,#20469,.T.);
#48815=EDGE_CURVE('',#38081,#38043,#20470,.T.);
#48816=EDGE_CURVE('',#38044,#38080,#20471,.T.);
#48817=EDGE_CURVE('',#38079,#38041,#20472,.T.);
#48818=EDGE_CURVE('',#38042,#38078,#20473,.T.);
#48819=EDGE_CURVE('',#38085,#38047,#20474,.T.);
#48820=EDGE_CURVE('',#38048,#38084,#20475,.T.);
#48821=EDGE_CURVE('',#38083,#38045,#20476,.T.);
#48822=EDGE_CURVE('',#38046,#38082,#20477,.T.);
#48823=EDGE_CURVE('',#38089,#38051,#20478,.T.);
#48824=EDGE_CURVE('',#38052,#38088,#20479,.T.);
#48825=EDGE_CURVE('',#38087,#38049,#20480,.T.);
#48826=EDGE_CURVE('',#38050,#38086,#20481,.T.);
#48827=EDGE_CURVE('',#38093,#38055,#20482,.T.);
#48828=EDGE_CURVE('',#38056,#38092,#20483,.T.);
#48829=EDGE_CURVE('',#38091,#38053,#20484,.T.);
#48830=EDGE_CURVE('',#38054,#38090,#20485,.T.);
#48831=EDGE_CURVE('',#38096,#38096,#20486,.T.);
#48832=EDGE_CURVE('',#38096,#38097,#28874,.T.);
#48833=EDGE_CURVE('',#38097,#38097,#20487,.T.);
#48834=EDGE_CURVE('',#38098,#38098,#20488,.T.);
#48835=EDGE_CURVE('',#38098,#38096,#28875,.T.);
#48836=EDGE_CURVE('',#38098,#38099,#28876,.T.);
#48837=EDGE_CURVE('',#38099,#38099,#20489,.T.);
#48838=EDGE_CURVE('',#38100,#38100,#20490,.T.);
#48839=EDGE_CURVE('',#38100,#38101,#28877,.T.);
#48840=EDGE_CURVE('',#38101,#38101,#20491,.T.);
#48841=EDGE_CURVE('',#38102,#38102,#20492,.T.);
#48842=EDGE_CURVE('',#38102,#38100,#28878,.T.);
#48843=EDGE_CURVE('',#38102,#38103,#28879,.T.);
#48844=EDGE_CURVE('',#38103,#38103,#20493,.T.);
#48845=EDGE_CURVE('',#38104,#38104,#20494,.T.);
#48846=EDGE_CURVE('',#38104,#38105,#28880,.T.);
#48847=EDGE_CURVE('',#38105,#38105,#20495,.T.);
#48848=EDGE_CURVE('',#38106,#38106,#20496,.T.);
#48849=EDGE_CURVE('',#38106,#38104,#28881,.T.);
#48850=EDGE_CURVE('',#38106,#38107,#28882,.T.);
#48851=EDGE_CURVE('',#38107,#38107,#20497,.T.);
#48852=EDGE_CURVE('',#38108,#38108,#20498,.T.);
#48853=EDGE_CURVE('',#38108,#38109,#28883,.T.);
#48854=EDGE_CURVE('',#38109,#38109,#20499,.T.);
#48855=EDGE_CURVE('',#38110,#38110,#20500,.T.);
#48856=EDGE_CURVE('',#38110,#38108,#28884,.T.);
#48857=EDGE_CURVE('',#38110,#38111,#28885,.T.);
#48858=EDGE_CURVE('',#38111,#38111,#20501,.T.);
#48859=EDGE_CURVE('',#38112,#38112,#20502,.T.);
#48860=EDGE_CURVE('',#38112,#38113,#28886,.T.);
#48861=EDGE_CURVE('',#38113,#38113,#20503,.T.);
#48862=EDGE_CURVE('',#38114,#38114,#20504,.T.);
#48863=EDGE_CURVE('',#38114,#38112,#28887,.T.);
#48864=EDGE_CURVE('',#38114,#38115,#28888,.T.);
#48865=EDGE_CURVE('',#38115,#38115,#20505,.T.);
#48866=EDGE_CURVE('',#38116,#38116,#20506,.T.);
#48867=EDGE_CURVE('',#38116,#38117,#28889,.T.);
#48868=EDGE_CURVE('',#38117,#38117,#20507,.T.);
#48869=EDGE_CURVE('',#38118,#38118,#20508,.T.);
#48870=EDGE_CURVE('',#38118,#38116,#28890,.T.);
#48871=EDGE_CURVE('',#38118,#38119,#28891,.T.);
#48872=EDGE_CURVE('',#38119,#38119,#20509,.T.);
#48873=EDGE_CURVE('',#38120,#38120,#20510,.T.);
#48874=EDGE_CURVE('',#38120,#38121,#28892,.T.);
#48875=EDGE_CURVE('',#38121,#38121,#20511,.T.);
#48876=EDGE_CURVE('',#38122,#38122,#20512,.T.);
#48877=EDGE_CURVE('',#38122,#38120,#28893,.T.);
#48878=EDGE_CURVE('',#38122,#38123,#28894,.T.);
#48879=EDGE_CURVE('',#38123,#38123,#20513,.T.);
#48880=EDGE_CURVE('',#38124,#38124,#20514,.T.);
#48881=EDGE_CURVE('',#38124,#38125,#28895,.T.);
#48882=EDGE_CURVE('',#38125,#38125,#20515,.T.);
#48883=EDGE_CURVE('',#38126,#38126,#20516,.T.);
#48884=EDGE_CURVE('',#38126,#38124,#28896,.T.);
#48885=EDGE_CURVE('',#38126,#38127,#28897,.T.);
#48886=EDGE_CURVE('',#38127,#38127,#20517,.T.);
#68422=ORIENTED_EDGE('',*,*,#48713,.T.);
#68423=ORIENTED_EDGE('',*,*,#48714,.T.);
#68424=ORIENTED_EDGE('',*,*,#48715,.T.);
#68425=ORIENTED_EDGE('',*,*,#48714,.F.);
#68426=ORIENTED_EDGE('',*,*,#48716,.F.);
#68427=ORIENTED_EDGE('',*,*,#48713,.F.);
#68428=ORIENTED_EDGE('',*,*,#48715,.F.);
#68429=ORIENTED_EDGE('',*,*,#48717,.T.);
#68430=ORIENTED_EDGE('',*,*,#48718,.T.);
#68431=ORIENTED_EDGE('',*,*,#48719,.T.);
#68432=ORIENTED_EDGE('',*,*,#48720,.T.);
#68433=ORIENTED_EDGE('',*,*,#48721,.T.);
#68434=ORIENTED_EDGE('',*,*,#48722,.F.);
#68435=ORIENTED_EDGE('',*,*,#48723,.F.);
#68436=ORIENTED_EDGE('',*,*,#48721,.F.);
#68437=ORIENTED_EDGE('',*,*,#48724,.T.);
#68438=ORIENTED_EDGE('',*,*,#48725,.T.);
#68439=ORIENTED_EDGE('',*,*,#48726,.T.);
#68440=ORIENTED_EDGE('',*,*,#48717,.F.);
#68441=ORIENTED_EDGE('',*,*,#48727,.T.);
#68442=ORIENTED_EDGE('',*,*,#48728,.T.);
#68443=ORIENTED_EDGE('',*,*,#48729,.T.);
#68444=ORIENTED_EDGE('',*,*,#48730,.T.);
#68445=ORIENTED_EDGE('',*,*,#48731,.T.);
#68446=ORIENTED_EDGE('',*,*,#48732,.T.);
#68447=ORIENTED_EDGE('',*,*,#48733,.T.);
#68448=ORIENTED_EDGE('',*,*,#48734,.T.);
#68449=ORIENTED_EDGE('',*,*,#48735,.T.);
#68450=ORIENTED_EDGE('',*,*,#48736,.T.);
#68451=ORIENTED_EDGE('',*,*,#48737,.T.);
#68452=ORIENTED_EDGE('',*,*,#48738,.T.);
#68453=ORIENTED_EDGE('',*,*,#48739,.T.);
#68454=ORIENTED_EDGE('',*,*,#48740,.T.);
#68455=ORIENTED_EDGE('',*,*,#48741,.T.);
#68456=ORIENTED_EDGE('',*,*,#48742,.T.);
#68457=ORIENTED_EDGE('',*,*,#48743,.T.);
#68458=ORIENTED_EDGE('',*,*,#48744,.T.);
#68459=ORIENTED_EDGE('',*,*,#48745,.T.);
#68460=ORIENTED_EDGE('',*,*,#48746,.T.);
#68461=ORIENTED_EDGE('',*,*,#48747,.T.);
#68462=ORIENTED_EDGE('',*,*,#48748,.T.);
#68463=ORIENTED_EDGE('',*,*,#48749,.T.);
#68464=ORIENTED_EDGE('',*,*,#48750,.T.);
#68465=ORIENTED_EDGE('',*,*,#48751,.T.);
#68466=ORIENTED_EDGE('',*,*,#48752,.T.);
#68467=ORIENTED_EDGE('',*,*,#48753,.T.);
#68468=ORIENTED_EDGE('',*,*,#48754,.T.);
#68469=ORIENTED_EDGE('',*,*,#48716,.T.);
#68470=ORIENTED_EDGE('',*,*,#48755,.T.);
#68471=ORIENTED_EDGE('',*,*,#48756,.T.);
#68472=ORIENTED_EDGE('',*,*,#48757,.T.);
#68473=ORIENTED_EDGE('',*,*,#48755,.F.);
#68474=ORIENTED_EDGE('',*,*,#48758,.F.);
#68475=ORIENTED_EDGE('',*,*,#48759,.T.);
#68476=ORIENTED_EDGE('',*,*,#48760,.T.);
#68477=ORIENTED_EDGE('',*,*,#48761,.T.);
#68478=ORIENTED_EDGE('',*,*,#48762,.T.);
#68479=ORIENTED_EDGE('',*,*,#48763,.T.);
#68480=ORIENTED_EDGE('',*,*,#48756,.F.);
#68481=ORIENTED_EDGE('',*,*,#48757,.F.);
#68482=ORIENTED_EDGE('',*,*,#48763,.F.);
#68483=ORIENTED_EDGE('',*,*,#48764,.T.);
#68484=ORIENTED_EDGE('',*,*,#48765,.T.);
#68485=ORIENTED_EDGE('',*,*,#48766,.T.);
#68486=ORIENTED_EDGE('',*,*,#48759,.F.);
#68487=ORIENTED_EDGE('',*,*,#48767,.T.);
#68488=ORIENTED_EDGE('',*,*,#48768,.T.);
#68489=ORIENTED_EDGE('',*,*,#48769,.T.);
#68490=ORIENTED_EDGE('',*,*,#48770,.T.);
#68491=ORIENTED_EDGE('',*,*,#48771,.T.);
#68492=ORIENTED_EDGE('',*,*,#48772,.T.);
#68493=ORIENTED_EDGE('',*,*,#48773,.T.);
#68494=ORIENTED_EDGE('',*,*,#48774,.T.);
#68495=ORIENTED_EDGE('',*,*,#48775,.T.);
#68496=ORIENTED_EDGE('',*,*,#48776,.T.);
#68497=ORIENTED_EDGE('',*,*,#48777,.T.);
#68498=ORIENTED_EDGE('',*,*,#48778,.T.);
#68499=ORIENTED_EDGE('',*,*,#48779,.T.);
#68500=ORIENTED_EDGE('',*,*,#48780,.T.);
#68501=ORIENTED_EDGE('',*,*,#48781,.T.);
#68502=ORIENTED_EDGE('',*,*,#48782,.T.);
#68503=ORIENTED_EDGE('',*,*,#48783,.T.);
#68504=ORIENTED_EDGE('',*,*,#48784,.T.);
#68505=ORIENTED_EDGE('',*,*,#48785,.T.);
#68506=ORIENTED_EDGE('',*,*,#48786,.T.);
#68507=ORIENTED_EDGE('',*,*,#48787,.T.);
#68508=ORIENTED_EDGE('',*,*,#48788,.T.);
#68509=ORIENTED_EDGE('',*,*,#48789,.T.);
#68510=ORIENTED_EDGE('',*,*,#48790,.T.);
#68511=ORIENTED_EDGE('',*,*,#48791,.T.);
#68512=ORIENTED_EDGE('',*,*,#48792,.T.);
#68513=ORIENTED_EDGE('',*,*,#48793,.T.);
#68514=ORIENTED_EDGE('',*,*,#48794,.T.);
#68515=ORIENTED_EDGE('',*,*,#48795,.T.);
#68516=ORIENTED_EDGE('',*,*,#48796,.T.);
#68517=ORIENTED_EDGE('',*,*,#48758,.T.);
#68518=ORIENTED_EDGE('',*,*,#48796,.F.);
#68519=ORIENTED_EDGE('',*,*,#48795,.F.);
#68520=ORIENTED_EDGE('',*,*,#48797,.F.);
#68521=ORIENTED_EDGE('',*,*,#48797,.T.);
#68522=ORIENTED_EDGE('',*,*,#48798,.T.);
#68523=ORIENTED_EDGE('',*,*,#48722,.T.);
#68524=ORIENTED_EDGE('',*,*,#48723,.T.);
#68525=ORIENTED_EDGE('',*,*,#48798,.F.);
#68526=ORIENTED_EDGE('',*,*,#48729,.F.);
#68527=ORIENTED_EDGE('',*,*,#48799,.F.);
#68528=ORIENTED_EDGE('',*,*,#48769,.F.);
#68529=ORIENTED_EDGE('',*,*,#48800,.F.);
#68530=ORIENTED_EDGE('',*,*,#48730,.F.);
#68531=ORIENTED_EDGE('',*,*,#48800,.T.);
#68532=ORIENTED_EDGE('',*,*,#48768,.F.);
#68533=ORIENTED_EDGE('',*,*,#48801,.T.);
#68534=ORIENTED_EDGE('',*,*,#48727,.F.);
#68535=ORIENTED_EDGE('',*,*,#48801,.F.);
#68536=ORIENTED_EDGE('',*,*,#48767,.F.);
#68537=ORIENTED_EDGE('',*,*,#48802,.F.);
#68538=ORIENTED_EDGE('',*,*,#48728,.F.);
#68539=ORIENTED_EDGE('',*,*,#48802,.T.);
#68540=ORIENTED_EDGE('',*,*,#48770,.F.);
#68541=ORIENTED_EDGE('',*,*,#48799,.T.);
#68542=ORIENTED_EDGE('',*,*,#48733,.F.);
#68543=ORIENTED_EDGE('',*,*,#48803,.F.);
#68544=ORIENTED_EDGE('',*,*,#48773,.F.);
#68545=ORIENTED_EDGE('',*,*,#48804,.F.);
#68546=ORIENTED_EDGE('',*,*,#48734,.F.);
#68547=ORIENTED_EDGE('',*,*,#48804,.T.);
#68548=ORIENTED_EDGE('',*,*,#48772,.F.);
#68549=ORIENTED_EDGE('',*,*,#48805,.T.);
#68550=ORIENTED_EDGE('',*,*,#48731,.F.);
#68551=ORIENTED_EDGE('',*,*,#48805,.F.);
#68552=ORIENTED_EDGE('',*,*,#48771,.F.);
#68553=ORIENTED_EDGE('',*,*,#48806,.F.);
#68554=ORIENTED_EDGE('',*,*,#48732,.F.);
#68555=ORIENTED_EDGE('',*,*,#48806,.T.);
#68556=ORIENTED_EDGE('',*,*,#48774,.F.);
#68557=ORIENTED_EDGE('',*,*,#48803,.T.);
#68558=ORIENTED_EDGE('',*,*,#48737,.F.);
#68559=ORIENTED_EDGE('',*,*,#48807,.F.);
#68560=ORIENTED_EDGE('',*,*,#48777,.F.);
#68561=ORIENTED_EDGE('',*,*,#48808,.F.);
#68562=ORIENTED_EDGE('',*,*,#48738,.F.);
#68563=ORIENTED_EDGE('',*,*,#48808,.T.);
#68564=ORIENTED_EDGE('',*,*,#48776,.F.);
#68565=ORIENTED_EDGE('',*,*,#48809,.T.);
#68566=ORIENTED_EDGE('',*,*,#48735,.F.);
#68567=ORIENTED_EDGE('',*,*,#48809,.F.);
#68568=ORIENTED_EDGE('',*,*,#48775,.F.);
#68569=ORIENTED_EDGE('',*,*,#48810,.F.);
#68570=ORIENTED_EDGE('',*,*,#48736,.F.);
#68571=ORIENTED_EDGE('',*,*,#48810,.T.);
#68572=ORIENTED_EDGE('',*,*,#48778,.F.);
#68573=ORIENTED_EDGE('',*,*,#48807,.T.);
#68574=ORIENTED_EDGE('',*,*,#48720,.F.);
#68575=ORIENTED_EDGE('',*,*,#48811,.F.);
#68576=ORIENTED_EDGE('',*,*,#48760,.F.);
#68577=ORIENTED_EDGE('',*,*,#48766,.F.);
#68578=ORIENTED_EDGE('',*,*,#48812,.F.);
#68579=ORIENTED_EDGE('',*,*,#48724,.F.);
#68580=ORIENTED_EDGE('',*,*,#48725,.F.);
#68581=ORIENTED_EDGE('',*,*,#48812,.T.);
#68582=ORIENTED_EDGE('',*,*,#48765,.F.);
#68583=ORIENTED_EDGE('',*,*,#48813,.T.);
#68584=ORIENTED_EDGE('',*,*,#48726,.F.);
#68585=ORIENTED_EDGE('',*,*,#48813,.F.);
#68586=ORIENTED_EDGE('',*,*,#48764,.F.);
#68587=ORIENTED_EDGE('',*,*,#48762,.F.);
#68588=ORIENTED_EDGE('',*,*,#48814,.F.);
#68589=ORIENTED_EDGE('',*,*,#48718,.F.);
#68590=ORIENTED_EDGE('',*,*,#48719,.F.);
#68591=ORIENTED_EDGE('',*,*,#48814,.T.);
#68592=ORIENTED_EDGE('',*,*,#48761,.F.);
#68593=ORIENTED_EDGE('',*,*,#48811,.T.);
#68594=ORIENTED_EDGE('',*,*,#48741,.F.);
#68595=ORIENTED_EDGE('',*,*,#48815,.F.);
#68596=ORIENTED_EDGE('',*,*,#48781,.F.);
#68597=ORIENTED_EDGE('',*,*,#48816,.F.);
#68598=ORIENTED_EDGE('',*,*,#48742,.F.);
#68599=ORIENTED_EDGE('',*,*,#48816,.T.);
#68600=ORIENTED_EDGE('',*,*,#48780,.F.);
#68601=ORIENTED_EDGE('',*,*,#48817,.T.);
#68602=ORIENTED_EDGE('',*,*,#48739,.F.);
#68603=ORIENTED_EDGE('',*,*,#48817,.F.);
#68604=ORIENTED_EDGE('',*,*,#48779,.F.);
#68605=ORIENTED_EDGE('',*,*,#48818,.F.);
#68606=ORIENTED_EDGE('',*,*,#48740,.F.);
#68607=ORIENTED_EDGE('',*,*,#48818,.T.);
#68608=ORIENTED_EDGE('',*,*,#48782,.F.);
#68609=ORIENTED_EDGE('',*,*,#48815,.T.);
#68610=ORIENTED_EDGE('',*,*,#48745,.F.);
#68611=ORIENTED_EDGE('',*,*,#48819,.F.);
#68612=ORIENTED_EDGE('',*,*,#48785,.F.);
#68613=ORIENTED_EDGE('',*,*,#48820,.F.);
#68614=ORIENTED_EDGE('',*,*,#48746,.F.);
#68615=ORIENTED_EDGE('',*,*,#48820,.T.);
#68616=ORIENTED_EDGE('',*,*,#48784,.F.);
#68617=ORIENTED_EDGE('',*,*,#48821,.T.);
#68618=ORIENTED_EDGE('',*,*,#48743,.F.);
#68619=ORIENTED_EDGE('',*,*,#48821,.F.);
#68620=ORIENTED_EDGE('',*,*,#48783,.F.);
#68621=ORIENTED_EDGE('',*,*,#48822,.F.);
#68622=ORIENTED_EDGE('',*,*,#48744,.F.);
#68623=ORIENTED_EDGE('',*,*,#48822,.T.);
#68624=ORIENTED_EDGE('',*,*,#48786,.F.);
#68625=ORIENTED_EDGE('',*,*,#48819,.T.);
#68626=ORIENTED_EDGE('',*,*,#48749,.F.);
#68627=ORIENTED_EDGE('',*,*,#48823,.F.);
#68628=ORIENTED_EDGE('',*,*,#48789,.F.);
#68629=ORIENTED_EDGE('',*,*,#48824,.F.);
#68630=ORIENTED_EDGE('',*,*,#48750,.F.);
#68631=ORIENTED_EDGE('',*,*,#48824,.T.);
#68632=ORIENTED_EDGE('',*,*,#48788,.F.);
#68633=ORIENTED_EDGE('',*,*,#48825,.T.);
#68634=ORIENTED_EDGE('',*,*,#48747,.F.);
#68635=ORIENTED_EDGE('',*,*,#48825,.F.);
#68636=ORIENTED_EDGE('',*,*,#48787,.F.);
#68637=ORIENTED_EDGE('',*,*,#48826,.F.);
#68638=ORIENTED_EDGE('',*,*,#48748,.F.);
#68639=ORIENTED_EDGE('',*,*,#48826,.T.);
#68640=ORIENTED_EDGE('',*,*,#48790,.F.);
#68641=ORIENTED_EDGE('',*,*,#48823,.T.);
#68642=ORIENTED_EDGE('',*,*,#48753,.F.);
#68643=ORIENTED_EDGE('',*,*,#48827,.F.);
#68644=ORIENTED_EDGE('',*,*,#48793,.F.);
#68645=ORIENTED_EDGE('',*,*,#48828,.F.);
#68646=ORIENTED_EDGE('',*,*,#48754,.F.);
#68647=ORIENTED_EDGE('',*,*,#48828,.T.);
#68648=ORIENTED_EDGE('',*,*,#48792,.F.);
#68649=ORIENTED_EDGE('',*,*,#48829,.T.);
#68650=ORIENTED_EDGE('',*,*,#48751,.F.);
#68651=ORIENTED_EDGE('',*,*,#48829,.F.);
#68652=ORIENTED_EDGE('',*,*,#48791,.F.);
#68653=ORIENTED_EDGE('',*,*,#48830,.F.);
#68654=ORIENTED_EDGE('',*,*,#48752,.F.);
#68655=ORIENTED_EDGE('',*,*,#48830,.T.);
#68656=ORIENTED_EDGE('',*,*,#48794,.F.);
#68657=ORIENTED_EDGE('',*,*,#48827,.T.);
#68658=ORIENTED_EDGE('',*,*,#48831,.T.);
#68659=ORIENTED_EDGE('',*,*,#48832,.T.);
#68660=ORIENTED_EDGE('',*,*,#48833,.T.);
#68661=ORIENTED_EDGE('',*,*,#48832,.F.);
#68662=ORIENTED_EDGE('',*,*,#48834,.F.);
#68663=ORIENTED_EDGE('',*,*,#48835,.T.);
#68664=ORIENTED_EDGE('',*,*,#48831,.F.);
#68665=ORIENTED_EDGE('',*,*,#48835,.F.);
#68666=ORIENTED_EDGE('',*,*,#48833,.F.);
#68667=ORIENTED_EDGE('',*,*,#48834,.T.);
#68668=ORIENTED_EDGE('',*,*,#48836,.T.);
#68669=ORIENTED_EDGE('',*,*,#48837,.T.);
#68670=ORIENTED_EDGE('',*,*,#48836,.F.);
#68671=ORIENTED_EDGE('',*,*,#48837,.F.);
#68672=ORIENTED_EDGE('',*,*,#48838,.T.);
#68673=ORIENTED_EDGE('',*,*,#48839,.T.);
#68674=ORIENTED_EDGE('',*,*,#48840,.T.);
#68675=ORIENTED_EDGE('',*,*,#48839,.F.);
#68676=ORIENTED_EDGE('',*,*,#48841,.F.);
#68677=ORIENTED_EDGE('',*,*,#48842,.T.);
#68678=ORIENTED_EDGE('',*,*,#48838,.F.);
#68679=ORIENTED_EDGE('',*,*,#48842,.F.);
#68680=ORIENTED_EDGE('',*,*,#48840,.F.);
#68681=ORIENTED_EDGE('',*,*,#48841,.T.);
#68682=ORIENTED_EDGE('',*,*,#48843,.T.);
#68683=ORIENTED_EDGE('',*,*,#48844,.T.);
#68684=ORIENTED_EDGE('',*,*,#48843,.F.);
#68685=ORIENTED_EDGE('',*,*,#48844,.F.);
#68686=ORIENTED_EDGE('',*,*,#48845,.T.);
#68687=ORIENTED_EDGE('',*,*,#48846,.T.);
#68688=ORIENTED_EDGE('',*,*,#48847,.T.);
#68689=ORIENTED_EDGE('',*,*,#48846,.F.);
#68690=ORIENTED_EDGE('',*,*,#48848,.F.);
#68691=ORIENTED_EDGE('',*,*,#48849,.T.);
#68692=ORIENTED_EDGE('',*,*,#48845,.F.);
#68693=ORIENTED_EDGE('',*,*,#48849,.F.);
#68694=ORIENTED_EDGE('',*,*,#48847,.F.);
#68695=ORIENTED_EDGE('',*,*,#48848,.T.);
#68696=ORIENTED_EDGE('',*,*,#48850,.T.);
#68697=ORIENTED_EDGE('',*,*,#48851,.T.);
#68698=ORIENTED_EDGE('',*,*,#48850,.F.);
#68699=ORIENTED_EDGE('',*,*,#48851,.F.);
#68700=ORIENTED_EDGE('',*,*,#48852,.T.);
#68701=ORIENTED_EDGE('',*,*,#48853,.T.);
#68702=ORIENTED_EDGE('',*,*,#48854,.T.);
#68703=ORIENTED_EDGE('',*,*,#48853,.F.);
#68704=ORIENTED_EDGE('',*,*,#48855,.F.);
#68705=ORIENTED_EDGE('',*,*,#48856,.T.);
#68706=ORIENTED_EDGE('',*,*,#48852,.F.);
#68707=ORIENTED_EDGE('',*,*,#48856,.F.);
#68708=ORIENTED_EDGE('',*,*,#48854,.F.);
#68709=ORIENTED_EDGE('',*,*,#48855,.T.);
#68710=ORIENTED_EDGE('',*,*,#48857,.T.);
#68711=ORIENTED_EDGE('',*,*,#48858,.T.);
#68712=ORIENTED_EDGE('',*,*,#48857,.F.);
#68713=ORIENTED_EDGE('',*,*,#48858,.F.);
#68714=ORIENTED_EDGE('',*,*,#48859,.T.);
#68715=ORIENTED_EDGE('',*,*,#48860,.T.);
#68716=ORIENTED_EDGE('',*,*,#48861,.T.);
#68717=ORIENTED_EDGE('',*,*,#48860,.F.);
#68718=ORIENTED_EDGE('',*,*,#48862,.F.);
#68719=ORIENTED_EDGE('',*,*,#48863,.T.);
#68720=ORIENTED_EDGE('',*,*,#48859,.F.);
#68721=ORIENTED_EDGE('',*,*,#48863,.F.);
#68722=ORIENTED_EDGE('',*,*,#48861,.F.);
#68723=ORIENTED_EDGE('',*,*,#48862,.T.);
#68724=ORIENTED_EDGE('',*,*,#48864,.T.);
#68725=ORIENTED_EDGE('',*,*,#48865,.T.);
#68726=ORIENTED_EDGE('',*,*,#48864,.F.);
#68727=ORIENTED_EDGE('',*,*,#48865,.F.);
#68728=ORIENTED_EDGE('',*,*,#48866,.T.);
#68729=ORIENTED_EDGE('',*,*,#48867,.T.);
#68730=ORIENTED_EDGE('',*,*,#48868,.T.);
#68731=ORIENTED_EDGE('',*,*,#48867,.F.);
#68732=ORIENTED_EDGE('',*,*,#48869,.F.);
#68733=ORIENTED_EDGE('',*,*,#48870,.T.);
#68734=ORIENTED_EDGE('',*,*,#48866,.F.);
#68735=ORIENTED_EDGE('',*,*,#48870,.F.);
#68736=ORIENTED_EDGE('',*,*,#48868,.F.);
#68737=ORIENTED_EDGE('',*,*,#48869,.T.);
#68738=ORIENTED_EDGE('',*,*,#48871,.T.);
#68739=ORIENTED_EDGE('',*,*,#48872,.T.);
#68740=ORIENTED_EDGE('',*,*,#48871,.F.);
#68741=ORIENTED_EDGE('',*,*,#48872,.F.);
#68742=ORIENTED_EDGE('',*,*,#48873,.T.);
#68743=ORIENTED_EDGE('',*,*,#48874,.T.);
#68744=ORIENTED_EDGE('',*,*,#48875,.T.);
#68745=ORIENTED_EDGE('',*,*,#48874,.F.);
#68746=ORIENTED_EDGE('',*,*,#48876,.F.);
#68747=ORIENTED_EDGE('',*,*,#48877,.T.);
#68748=ORIENTED_EDGE('',*,*,#48873,.F.);
#68749=ORIENTED_EDGE('',*,*,#48877,.F.);
#68750=ORIENTED_EDGE('',*,*,#48875,.F.);
#68751=ORIENTED_EDGE('',*,*,#48876,.T.);
#68752=ORIENTED_EDGE('',*,*,#48878,.T.);
#68753=ORIENTED_EDGE('',*,*,#48879,.T.);
#68754=ORIENTED_EDGE('',*,*,#48878,.F.);
#68755=ORIENTED_EDGE('',*,*,#48879,.F.);
#68756=ORIENTED_EDGE('',*,*,#48880,.T.);
#68757=ORIENTED_EDGE('',*,*,#48881,.T.);
#68758=ORIENTED_EDGE('',*,*,#48882,.T.);
#68759=ORIENTED_EDGE('',*,*,#48881,.F.);
#68760=ORIENTED_EDGE('',*,*,#48883,.F.);
#68761=ORIENTED_EDGE('',*,*,#48884,.T.);
#68762=ORIENTED_EDGE('',*,*,#48880,.F.);
#68763=ORIENTED_EDGE('',*,*,#48884,.F.);
#68764=ORIENTED_EDGE('',*,*,#48882,.F.);
#68765=ORIENTED_EDGE('',*,*,#48883,.T.);
#68766=ORIENTED_EDGE('',*,*,#48885,.T.);
#68767=ORIENTED_EDGE('',*,*,#48886,.T.);
#68768=ORIENTED_EDGE('',*,*,#48885,.F.);
#68769=ORIENTED_EDGE('',*,*,#48886,.F.);
#87829=CYLINDRICAL_SURFACE('',#98863,1.6);
#87830=CYLINDRICAL_SURFACE('',#98888,2.4);
#87831=CYLINDRICAL_SURFACE('',#98918,0.525);
#87832=CYLINDRICAL_SURFACE('',#98922,0.525);
#87833=CYLINDRICAL_SURFACE('',#98926,0.525);
#87834=CYLINDRICAL_SURFACE('',#98930,0.525);
#87835=CYLINDRICAL_SURFACE('',#98934,0.525);
#87836=CYLINDRICAL_SURFACE('',#98938,0.525);
#87837=CYLINDRICAL_SURFACE('',#98942,0.525);
#87838=CYLINDRICAL_SURFACE('',#98946,0.525);
#87839=CYLINDRICAL_SURFACE('',#98950,0.525);
#87840=CYLINDRICAL_SURFACE('',#98954,0.525);
#87841=CYLINDRICAL_SURFACE('',#98958,0.525);
#87842=CYLINDRICAL_SURFACE('',#98962,0.525);
#87843=CYLINDRICAL_SURFACE('',#98966,0.525);
#87844=CYLINDRICAL_SURFACE('',#98970,0.525);
#87845=CYLINDRICAL_SURFACE('',#98974,0.525);
#87846=CYLINDRICAL_SURFACE('',#98978,0.525);
#87847=CYLINDRICAL_SURFACE('',#98982,0.5);
#87848=CYLINDRICAL_SURFACE('',#98991,0.5);
#87849=CYLINDRICAL_SURFACE('',#99000,0.5);
#87850=CYLINDRICAL_SURFACE('',#99009,0.5);
#87851=CYLINDRICAL_SURFACE('',#99018,0.5);
#87852=CYLINDRICAL_SURFACE('',#99027,0.5);
#87853=CYLINDRICAL_SURFACE('',#99036,0.5);
#87854=CYLINDRICAL_SURFACE('',#99045,0.5);
#90697=ADVANCED_FACE('',(#8233),#1858,.T.);
#90698=ADVANCED_FACE('',(#8234,#5193),#5650,.F.);
#90699=ADVANCED_FACE('',(#8235,#5194,#5195,#5196,#5197,#5198,#5199,#5200),
#87829,.F.);
#90700=ADVANCED_FACE('',(#8236),#1859,.T.);
#90701=ADVANCED_FACE('',(#8237,#5201,#5202,#5203,#5204,#5205,#5206,#5207),
#87830,.T.);
#90702=ADVANCED_FACE('',(#8238),#1860,.T.);
#90703=ADVANCED_FACE('',(#8239,#5208),#5651,.T.);
#90704=ADVANCED_FACE('',(#8240),#1861,.T.);
#90705=ADVANCED_FACE('',(#8241),#5652,.F.);
#90706=ADVANCED_FACE('',(#8242),#87831,.F.);
#90707=ADVANCED_FACE('',(#8243),#5653,.T.);
#90708=ADVANCED_FACE('',(#8244),#87832,.F.);
#90709=ADVANCED_FACE('',(#8245),#5654,.F.);
#90710=ADVANCED_FACE('',(#8246),#87833,.F.);
#90711=ADVANCED_FACE('',(#8247),#5655,.T.);
#90712=ADVANCED_FACE('',(#8248),#87834,.F.);
#90713=ADVANCED_FACE('',(#8249),#5656,.F.);
#90714=ADVANCED_FACE('',(#8250),#87835,.F.);
#90715=ADVANCED_FACE('',(#8251),#5657,.T.);
#90716=ADVANCED_FACE('',(#8252),#87836,.F.);
#90717=ADVANCED_FACE('',(#8253),#5658,.F.);
#90718=ADVANCED_FACE('',(#8254),#87837,.F.);
#90719=ADVANCED_FACE('',(#8255),#5659,.T.);
#90720=ADVANCED_FACE('',(#8256),#87838,.F.);
#90721=ADVANCED_FACE('',(#8257),#5660,.F.);
#90722=ADVANCED_FACE('',(#8258),#87839,.F.);
#90723=ADVANCED_FACE('',(#8259),#5661,.T.);
#90724=ADVANCED_FACE('',(#8260),#87840,.F.);
#90725=ADVANCED_FACE('',(#8261),#5662,.F.);
#90726=ADVANCED_FACE('',(#8262),#87841,.F.);
#90727=ADVANCED_FACE('',(#8263),#5663,.T.);
#90728=ADVANCED_FACE('',(#8264),#87842,.F.);
#90729=ADVANCED_FACE('',(#8265),#5664,.F.);
#90730=ADVANCED_FACE('',(#8266),#87843,.F.);
#90731=ADVANCED_FACE('',(#8267),#5665,.T.);
#90732=ADVANCED_FACE('',(#8268),#87844,.F.);
#90733=ADVANCED_FACE('',(#8269),#5666,.F.);
#90734=ADVANCED_FACE('',(#8270),#87845,.F.);
#90735=ADVANCED_FACE('',(#8271),#5667,.T.);
#90736=ADVANCED_FACE('',(#8272),#87846,.F.);
#90737=ADVANCED_FACE('',(#8273),#4861,.T.);
#90738=ADVANCED_FACE('',(#8274),#87847,.T.);
#90739=ADVANCED_FACE('',(#8275),#5668,.F.);
#90740=ADVANCED_FACE('',(#8276),#4862,.T.);
#90741=ADVANCED_FACE('',(#8277),#5669,.T.);
#90742=ADVANCED_FACE('',(#8278),#4863,.T.);
#90743=ADVANCED_FACE('',(#8279),#87848,.T.);
#90744=ADVANCED_FACE('',(#8280),#5670,.F.);
#90745=ADVANCED_FACE('',(#8281),#4864,.T.);
#90746=ADVANCED_FACE('',(#8282),#5671,.T.);
#90747=ADVANCED_FACE('',(#8283),#4865,.T.);
#90748=ADVANCED_FACE('',(#8284),#87849,.T.);
#90749=ADVANCED_FACE('',(#8285),#5672,.F.);
#90750=ADVANCED_FACE('',(#8286),#4866,.T.);
#90751=ADVANCED_FACE('',(#8287),#5673,.T.);
#90752=ADVANCED_FACE('',(#8288),#4867,.T.);
#90753=ADVANCED_FACE('',(#8289),#87850,.T.);
#90754=ADVANCED_FACE('',(#8290),#5674,.F.);
#90755=ADVANCED_FACE('',(#8291),#4868,.T.);
#90756=ADVANCED_FACE('',(#8292),#5675,.T.);
#90757=ADVANCED_FACE('',(#8293),#4869,.T.);
#90758=ADVANCED_FACE('',(#8294),#87851,.T.);
#90759=ADVANCED_FACE('',(#8295),#5676,.F.);
#90760=ADVANCED_FACE('',(#8296),#4870,.T.);
#90761=ADVANCED_FACE('',(#8297),#5677,.T.);
#90762=ADVANCED_FACE('',(#8298),#4871,.T.);
#90763=ADVANCED_FACE('',(#8299),#87852,.T.);
#90764=ADVANCED_FACE('',(#8300),#5678,.F.);
#90765=ADVANCED_FACE('',(#8301),#4872,.T.);
#90766=ADVANCED_FACE('',(#8302),#5679,.T.);
#90767=ADVANCED_FACE('',(#8303),#4873,.T.);
#90768=ADVANCED_FACE('',(#8304),#87853,.T.);
#90769=ADVANCED_FACE('',(#8305),#5680,.F.);
#90770=ADVANCED_FACE('',(#8306),#4874,.T.);
#90771=ADVANCED_FACE('',(#8307),#5681,.T.);
#90772=ADVANCED_FACE('',(#8308),#4875,.T.);
#90773=ADVANCED_FACE('',(#8309),#87854,.T.);
#90774=ADVANCED_FACE('',(#8310),#5682,.F.);
#90775=ADVANCED_FACE('',(#8311),#4876,.T.);
#90776=ADVANCED_FACE('',(#8312),#5683,.T.);
#94636=CLOSED_SHELL('',(#90697,#90698,#90699,#90700,#90701,#90702,#90703,
#90704,#90705,#90706,#90707,#90708,#90709,#90710,#90711,#90712,#90713,#90714,
#90715,#90716,#90717,#90718,#90719,#90720,#90721,#90722,#90723,#90724,#90725,
#90726,#90727,#90728,#90729,#90730,#90731,#90732,#90733,#90734,#90735,#90736));
#94637=CLOSED_SHELL('',(#90737,#90738,#90739,#90740,#90741));
#94638=CLOSED_SHELL('',(#90742,#90743,#90744,#90745,#90746));
#94639=CLOSED_SHELL('',(#90747,#90748,#90749,#90750,#90751));
#94640=CLOSED_SHELL('',(#90752,#90753,#90754,#90755,#90756));
#94641=CLOSED_SHELL('',(#90757,#90758,#90759,#90760,#90761));
#94642=CLOSED_SHELL('',(#90762,#90763,#90764,#90765,#90766));
#94643=CLOSED_SHELL('',(#90767,#90768,#90769,#90770,#90771));
#94644=CLOSED_SHELL('',(#90772,#90773,#90774,#90775,#90776));
#98856=AXIS2_PLACEMENT_3D('',#358160,#115270,#115271);
#98857=AXIS2_PLACEMENT_3D('',#358161,#115272,#115273);
#98858=AXIS2_PLACEMENT_3D('',#358163,#115274,#115275);
#98859=AXIS2_PLACEMENT_3D('',#358165,#115276,#115277);
#98860=AXIS2_PLACEMENT_3D('',#358166,#115278,#115279);
#98861=AXIS2_PLACEMENT_3D('',#358167,#115280,#115281);
#98862=AXIS2_PLACEMENT_3D('',#358169,#115282,#115283);
#98863=AXIS2_PLACEMENT_3D('',#358170,#115284,#115285);
#98864=AXIS2_PLACEMENT_3D('',#358174,#115287,#115288);
#98865=AXIS2_PLACEMENT_3D('',#358178,#115290,#115291);
#98866=AXIS2_PLACEMENT_3D('',#358182,#115293,#115294);
#98867=AXIS2_PLACEMENT_3D('',#358183,#115295,#115296);
#98868=AXIS2_PLACEMENT_3D('',#358185,#115297,#115298);
#98869=AXIS2_PLACEMENT_3D('',#358188,#115300,#115301);
#98870=AXIS2_PLACEMENT_3D('',#358191,#115302,#115303);
#98871=AXIS2_PLACEMENT_3D('',#358195,#115305,#115306);
#98872=AXIS2_PLACEMENT_3D('',#358199,#115308,#115309);
#98873=AXIS2_PLACEMENT_3D('',#358203,#115311,#115312);
#98874=AXIS2_PLACEMENT_3D('',#358207,#115314,#115315);
#98875=AXIS2_PLACEMENT_3D('',#358211,#115317,#115318);
#98876=AXIS2_PLACEMENT_3D('',#358215,#115320,#115321);
#98877=AXIS2_PLACEMENT_3D('',#358219,#115323,#115324);
#98878=AXIS2_PLACEMENT_3D('',#358223,#115326,#115327);
#98879=AXIS2_PLACEMENT_3D('',#358227,#115329,#115330);
#98880=AXIS2_PLACEMENT_3D('',#358231,#115332,#115333);
#98881=AXIS2_PLACEMENT_3D('',#358235,#115335,#115336);
#98882=AXIS2_PLACEMENT_3D('',#358239,#115338,#115339);
#98883=AXIS2_PLACEMENT_3D('',#358243,#115341,#115342);
#98884=AXIS2_PLACEMENT_3D('',#358245,#115344,#115345);
#98885=AXIS2_PLACEMENT_3D('',#358247,#115346,#115347);
#98886=AXIS2_PLACEMENT_3D('',#358249,#115348,#115349);
#98887=AXIS2_PLACEMENT_3D('',#358250,#115350,#115351);
#98888=AXIS2_PLACEMENT_3D('',#358251,#115352,#115353);
#98889=AXIS2_PLACEMENT_3D('',#358253,#115354,#115355);
#98890=AXIS2_PLACEMENT_3D('',#358257,#115357,#115358);
#98891=AXIS2_PLACEMENT_3D('',#358261,#115360,#115361);
#98892=AXIS2_PLACEMENT_3D('',#358264,#115363,#115364);
#98893=AXIS2_PLACEMENT_3D('',#358267,#115366,#115367);
#98894=AXIS2_PLACEMENT_3D('',#358270,#115368,#115369);
#98895=AXIS2_PLACEMENT_3D('',#358274,#115371,#115372);
#98896=AXIS2_PLACEMENT_3D('',#358278,#115374,#115375);
#98897=AXIS2_PLACEMENT_3D('',#358282,#115377,#115378);
#98898=AXIS2_PLACEMENT_3D('',#358286,#115380,#115381);
#98899=AXIS2_PLACEMENT_3D('',#358290,#115383,#115384);
#98900=AXIS2_PLACEMENT_3D('',#358294,#115386,#115387);
#98901=AXIS2_PLACEMENT_3D('',#358298,#115389,#115390);
#98902=AXIS2_PLACEMENT_3D('',#358302,#115392,#115393);
#98903=AXIS2_PLACEMENT_3D('',#358306,#115395,#115396);
#98904=AXIS2_PLACEMENT_3D('',#358310,#115398,#115399);
#98905=AXIS2_PLACEMENT_3D('',#358314,#115401,#115402);
#98906=AXIS2_PLACEMENT_3D('',#358318,#115404,#115405);
#98907=AXIS2_PLACEMENT_3D('',#358322,#115407,#115408);
#98908=AXIS2_PLACEMENT_3D('',#358324,#115410,#115411);
#98909=AXIS2_PLACEMENT_3D('',#358326,#115412,#115413);
#98910=AXIS2_PLACEMENT_3D('',#358327,#115414,#115415);
#98911=AXIS2_PLACEMENT_3D('',#358328,#115416,#115417);
#98912=AXIS2_PLACEMENT_3D('',#358330,#115418,#115419);
#98913=AXIS2_PLACEMENT_3D('',#358331,#115420,#115421);
#98914=AXIS2_PLACEMENT_3D('',#358332,#115422,#115423);
#98915=AXIS2_PLACEMENT_3D('',#358333,#115424,#115425);
#98916=AXIS2_PLACEMENT_3D('',#358334,#115426,#115427);
#98917=AXIS2_PLACEMENT_3D('',#358335,#115428,#115429);
#98918=AXIS2_PLACEMENT_3D('',#358336,#115430,#115431);
#98919=AXIS2_PLACEMENT_3D('',#358337,#115432,#115433);
#98920=AXIS2_PLACEMENT_3D('',#358338,#115434,#115435);
#98921=AXIS2_PLACEMENT_3D('',#358339,#115436,#115437);
#98922=AXIS2_PLACEMENT_3D('',#358340,#115438,#115439);
#98923=AXIS2_PLACEMENT_3D('',#358341,#115440,#115441);
#98924=AXIS2_PLACEMENT_3D('',#358342,#115442,#115443);
#98925=AXIS2_PLACEMENT_3D('',#358343,#115444,#115445);
#98926=AXIS2_PLACEMENT_3D('',#358344,#115446,#115447);
#98927=AXIS2_PLACEMENT_3D('',#358345,#115448,#115449);
#98928=AXIS2_PLACEMENT_3D('',#358346,#115450,#115451);
#98929=AXIS2_PLACEMENT_3D('',#358347,#115452,#115453);
#98930=AXIS2_PLACEMENT_3D('',#358348,#115454,#115455);
#98931=AXIS2_PLACEMENT_3D('',#358349,#115456,#115457);
#98932=AXIS2_PLACEMENT_3D('',#358350,#115458,#115459);
#98933=AXIS2_PLACEMENT_3D('',#358351,#115460,#115461);
#98934=AXIS2_PLACEMENT_3D('',#358352,#115462,#115463);
#98935=AXIS2_PLACEMENT_3D('',#358353,#115464,#115465);
#98936=AXIS2_PLACEMENT_3D('',#358354,#115466,#115467);
#98937=AXIS2_PLACEMENT_3D('',#358355,#115468,#115469);
#98938=AXIS2_PLACEMENT_3D('',#358356,#115470,#115471);
#98939=AXIS2_PLACEMENT_3D('',#358357,#115472,#115473);
#98940=AXIS2_PLACEMENT_3D('',#358358,#115474,#115475);
#98941=AXIS2_PLACEMENT_3D('',#358359,#115476,#115477);
#98942=AXIS2_PLACEMENT_3D('',#358360,#115478,#115479);
#98943=AXIS2_PLACEMENT_3D('',#358361,#115480,#115481);
#98944=AXIS2_PLACEMENT_3D('',#358362,#115482,#115483);
#98945=AXIS2_PLACEMENT_3D('',#358363,#115484,#115485);
#98946=AXIS2_PLACEMENT_3D('',#358364,#115486,#115487);
#98947=AXIS2_PLACEMENT_3D('',#358365,#115488,#115489);
#98948=AXIS2_PLACEMENT_3D('',#358366,#115490,#115491);
#98949=AXIS2_PLACEMENT_3D('',#358367,#115492,#115493);
#98950=AXIS2_PLACEMENT_3D('',#358368,#115494,#115495);
#98951=AXIS2_PLACEMENT_3D('',#358369,#115496,#115497);
#98952=AXIS2_PLACEMENT_3D('',#358370,#115498,#115499);
#98953=AXIS2_PLACEMENT_3D('',#358371,#115500,#115501);
#98954=AXIS2_PLACEMENT_3D('',#358372,#115502,#115503);
#98955=AXIS2_PLACEMENT_3D('',#358373,#115504,#115505);
#98956=AXIS2_PLACEMENT_3D('',#358374,#115506,#115507);
#98957=AXIS2_PLACEMENT_3D('',#358375,#115508,#115509);
#98958=AXIS2_PLACEMENT_3D('',#358376,#115510,#115511);
#98959=AXIS2_PLACEMENT_3D('',#358377,#115512,#115513);
#98960=AXIS2_PLACEMENT_3D('',#358378,#115514,#115515);
#98961=AXIS2_PLACEMENT_3D('',#358379,#115516,#115517);
#98962=AXIS2_PLACEMENT_3D('',#358380,#115518,#115519);
#98963=AXIS2_PLACEMENT_3D('',#358381,#115520,#115521);
#98964=AXIS2_PLACEMENT_3D('',#358382,#115522,#115523);
#98965=AXIS2_PLACEMENT_3D('',#358383,#115524,#115525);
#98966=AXIS2_PLACEMENT_3D('',#358384,#115526,#115527);
#98967=AXIS2_PLACEMENT_3D('',#358385,#115528,#115529);
#98968=AXIS2_PLACEMENT_3D('',#358386,#115530,#115531);
#98969=AXIS2_PLACEMENT_3D('',#358387,#115532,#115533);
#98970=AXIS2_PLACEMENT_3D('',#358388,#115534,#115535);
#98971=AXIS2_PLACEMENT_3D('',#358389,#115536,#115537);
#98972=AXIS2_PLACEMENT_3D('',#358390,#115538,#115539);
#98973=AXIS2_PLACEMENT_3D('',#358391,#115540,#115541);
#98974=AXIS2_PLACEMENT_3D('',#358392,#115542,#115543);
#98975=AXIS2_PLACEMENT_3D('',#358393,#115544,#115545);
#98976=AXIS2_PLACEMENT_3D('',#358394,#115546,#115547);
#98977=AXIS2_PLACEMENT_3D('',#358395,#115548,#115549);
#98978=AXIS2_PLACEMENT_3D('',#358396,#115550,#115551);
#98979=AXIS2_PLACEMENT_3D('',#358397,#115552,#115553);
#98980=AXIS2_PLACEMENT_3D('',#358399,#115554,#115555);
#98981=AXIS2_PLACEMENT_3D('',#358402,#115557,#115558);
#98982=AXIS2_PLACEMENT_3D('',#358403,#115559,#115560);
#98983=AXIS2_PLACEMENT_3D('',#358405,#115561,#115562);
#98984=AXIS2_PLACEMENT_3D('',#358407,#115564,#115565);
#98985=AXIS2_PLACEMENT_3D('',#358408,#115566,#115567);
#98986=AXIS2_PLACEMENT_3D('',#358411,#115569,#115570);
#98987=AXIS2_PLACEMENT_3D('',#358412,#115571,#115572);
#98988=AXIS2_PLACEMENT_3D('',#358413,#115573,#115574);
#98989=AXIS2_PLACEMENT_3D('',#358415,#115575,#115576);
#98990=AXIS2_PLACEMENT_3D('',#358418,#115578,#115579);
#98991=AXIS2_PLACEMENT_3D('',#358419,#115580,#115581);
#98992=AXIS2_PLACEMENT_3D('',#358421,#115582,#115583);
#98993=AXIS2_PLACEMENT_3D('',#358423,#115585,#115586);
#98994=AXIS2_PLACEMENT_3D('',#358424,#115587,#115588);
#98995=AXIS2_PLACEMENT_3D('',#358427,#115590,#115591);
#98996=AXIS2_PLACEMENT_3D('',#358428,#115592,#115593);
#98997=AXIS2_PLACEMENT_3D('',#358429,#115594,#115595);
#98998=AXIS2_PLACEMENT_3D('',#358431,#115596,#115597);
#98999=AXIS2_PLACEMENT_3D('',#358434,#115599,#115600);
#99000=AXIS2_PLACEMENT_3D('',#358435,#115601,#115602);
#99001=AXIS2_PLACEMENT_3D('',#358437,#115603,#115604);
#99002=AXIS2_PLACEMENT_3D('',#358439,#115606,#115607);
#99003=AXIS2_PLACEMENT_3D('',#358440,#115608,#115609);
#99004=AXIS2_PLACEMENT_3D('',#358443,#115611,#115612);
#99005=AXIS2_PLACEMENT_3D('',#358444,#115613,#115614);
#99006=AXIS2_PLACEMENT_3D('',#358445,#115615,#115616);
#99007=AXIS2_PLACEMENT_3D('',#358447,#115617,#115618);
#99008=AXIS2_PLACEMENT_3D('',#358450,#115620,#115621);
#99009=AXIS2_PLACEMENT_3D('',#358451,#115622,#115623);
#99010=AXIS2_PLACEMENT_3D('',#358453,#115624,#115625);
#99011=AXIS2_PLACEMENT_3D('',#358455,#115627,#115628);
#99012=AXIS2_PLACEMENT_3D('',#358456,#115629,#115630);
#99013=AXIS2_PLACEMENT_3D('',#358459,#115632,#115633);
#99014=AXIS2_PLACEMENT_3D('',#358460,#115634,#115635);
#99015=AXIS2_PLACEMENT_3D('',#358461,#115636,#115637);
#99016=AXIS2_PLACEMENT_3D('',#358463,#115638,#115639);
#99017=AXIS2_PLACEMENT_3D('',#358466,#115641,#115642);
#99018=AXIS2_PLACEMENT_3D('',#358467,#115643,#115644);
#99019=AXIS2_PLACEMENT_3D('',#358469,#115645,#115646);
#99020=AXIS2_PLACEMENT_3D('',#358471,#115648,#115649);
#99021=AXIS2_PLACEMENT_3D('',#358472,#115650,#115651);
#99022=AXIS2_PLACEMENT_3D('',#358475,#115653,#115654);
#99023=AXIS2_PLACEMENT_3D('',#358476,#115655,#115656);
#99024=AXIS2_PLACEMENT_3D('',#358477,#115657,#115658);
#99025=AXIS2_PLACEMENT_3D('',#358479,#115659,#115660);
#99026=AXIS2_PLACEMENT_3D('',#358482,#115662,#115663);
#99027=AXIS2_PLACEMENT_3D('',#358483,#115664,#115665);
#99028=AXIS2_PLACEMENT_3D('',#358485,#115666,#115667);
#99029=AXIS2_PLACEMENT_3D('',#358487,#115669,#115670);
#99030=AXIS2_PLACEMENT_3D('',#358488,#115671,#115672);
#99031=AXIS2_PLACEMENT_3D('',#358491,#115674,#115675);
#99032=AXIS2_PLACEMENT_3D('',#358492,#115676,#115677);
#99033=AXIS2_PLACEMENT_3D('',#358493,#115678,#115679);
#99034=AXIS2_PLACEMENT_3D('',#358495,#115680,#115681);
#99035=AXIS2_PLACEMENT_3D('',#358498,#115683,#115684);
#99036=AXIS2_PLACEMENT_3D('',#358499,#115685,#115686);
#99037=AXIS2_PLACEMENT_3D('',#358501,#115687,#115688);
#99038=AXIS2_PLACEMENT_3D('',#358503,#115690,#115691);
#99039=AXIS2_PLACEMENT_3D('',#358504,#115692,#115693);
#99040=AXIS2_PLACEMENT_3D('',#358507,#115695,#115696);
#99041=AXIS2_PLACEMENT_3D('',#358508,#115697,#115698);
#99042=AXIS2_PLACEMENT_3D('',#358509,#115699,#115700);
#99043=AXIS2_PLACEMENT_3D('',#358511,#115701,#115702);
#99044=AXIS2_PLACEMENT_3D('',#358514,#115704,#115705);
#99045=AXIS2_PLACEMENT_3D('',#358515,#115706,#115707);
#99046=AXIS2_PLACEMENT_3D('',#358517,#115708,#115709);
#99047=AXIS2_PLACEMENT_3D('',#358519,#115711,#115712);
#99048=AXIS2_PLACEMENT_3D('',#358520,#115713,#115714);
#99049=AXIS2_PLACEMENT_3D('',#358523,#115716,#115717);
#99050=AXIS2_PLACEMENT_3D('',#358524,#115718,#115719);
#115270=DIRECTION('axis',(0.,0.,1.));
#115271=DIRECTION('refdir',(1.,0.,0.));
#115272=DIRECTION('center_axis',(0.,0.,1.));
#115273=DIRECTION('ref_axis',(1.,0.,0.));
#115274=DIRECTION('center_axis',(0.,0.,-1.));
#115275=DIRECTION('ref_axis',(1.,0.,0.));
#115276=DIRECTION('center_axis',(1.22464679914735E-16,-1.,0.));
#115277=DIRECTION('ref_axis',(-1.,-1.22464679914735E-16,0.));
#115278=DIRECTION('center_axis',(0.,0.,1.));
#115279=DIRECTION('ref_axis',(1.,0.,0.));
#115280=DIRECTION('center_axis',(0.,0.,1.));
#115281=DIRECTION('ref_axis',(1.,0.,0.));
#115282=DIRECTION('center_axis',(0.,0.,1.));
#115283=DIRECTION('ref_axis',(1.,0.,0.));
#115284=DIRECTION('center_axis',(0.,0.,1.));
#115285=DIRECTION('ref_axis',(1.,0.,0.));
#115286=DIRECTION('',(0.,0.,1.));
#115287=DIRECTION('center_axis',(0.,0.,1.));
#115288=DIRECTION('ref_axis',(1.,0.,0.));
#115289=DIRECTION('',(0.,0.,1.));
#115290=DIRECTION('center_axis',(0.,0.,-1.));
#115291=DIRECTION('ref_axis',(1.,0.,0.));
#115292=DIRECTION('',(0.,0.,1.));
#115293=DIRECTION('center_axis',(0.,0.,-1.));
#115294=DIRECTION('ref_axis',(1.,0.,0.));
#115295=DIRECTION('center_axis',(0.,0.,-1.));
#115296=DIRECTION('ref_axis',(1.,0.,0.));
#115297=DIRECTION('center_axis',(0.,0.,-1.));
#115298=DIRECTION('ref_axis',(1.,0.,0.));
#115299=DIRECTION('',(0.,0.,-1.));
#115300=DIRECTION('center_axis',(0.,0.,1.));
#115301=DIRECTION('ref_axis',(1.,0.,0.));
#115302=DIRECTION('center_axis',(0.,0.,1.));
#115303=DIRECTION('ref_axis',(1.,0.,0.));
#115304=DIRECTION('',(0.,0.,1.));
#115305=DIRECTION('center_axis',(0.,0.,-1.));
#115306=DIRECTION('ref_axis',(1.,0.,0.));
#115307=DIRECTION('',(0.,0.,-1.));
#115308=DIRECTION('center_axis',(0.,0.,1.));
#115309=DIRECTION('ref_axis',(1.,0.,0.));
#115310=DIRECTION('',(0.,0.,1.));
#115311=DIRECTION('center_axis',(0.,0.,-1.));
#115312=DIRECTION('ref_axis',(1.,0.,0.));
#115313=DIRECTION('',(0.,0.,-1.));
#115314=DIRECTION('center_axis',(0.,0.,1.));
#115315=DIRECTION('ref_axis',(1.,0.,0.));
#115316=DIRECTION('',(0.,0.,1.));
#115317=DIRECTION('center_axis',(0.,0.,-1.));
#115318=DIRECTION('ref_axis',(1.,0.,0.));
#115319=DIRECTION('',(0.,0.,-1.));
#115320=DIRECTION('center_axis',(0.,0.,1.));
#115321=DIRECTION('ref_axis',(1.,0.,0.));
#115322=DIRECTION('',(0.,0.,1.));
#115323=DIRECTION('center_axis',(0.,0.,-1.));
#115324=DIRECTION('ref_axis',(1.,0.,0.));
#115325=DIRECTION('',(0.,0.,-1.));
#115326=DIRECTION('center_axis',(0.,0.,1.));
#115327=DIRECTION('ref_axis',(1.,0.,0.));
#115328=DIRECTION('',(0.,0.,1.));
#115329=DIRECTION('center_axis',(0.,0.,-1.));
#115330=DIRECTION('ref_axis',(1.,0.,0.));
#115331=DIRECTION('',(0.,0.,-1.));
#115332=DIRECTION('center_axis',(0.,0.,1.));
#115333=DIRECTION('ref_axis',(1.,0.,0.));
#115334=DIRECTION('',(0.,0.,1.));
#115335=DIRECTION('center_axis',(0.,0.,-1.));
#115336=DIRECTION('ref_axis',(1.,0.,0.));
#115337=DIRECTION('',(0.,0.,-1.));
#115338=DIRECTION('center_axis',(0.,0.,1.));
#115339=DIRECTION('ref_axis',(1.,0.,0.));
#115340=DIRECTION('',(0.,0.,1.));
#115341=DIRECTION('center_axis',(0.,0.,-1.));
#115342=DIRECTION('ref_axis',(1.,0.,0.));
#115343=DIRECTION('',(0.,0.,-1.));
#115344=DIRECTION('center_axis',(0.,0.,-1.));
#115345=DIRECTION('ref_axis',(-1.,0.,0.));
#115346=DIRECTION('center_axis',(-1.22464679914735E-16,-1.,0.));
#115347=DIRECTION('ref_axis',(1.,-1.22464679914735E-16,0.));
#115348=DIRECTION('center_axis',(0.,0.,-1.));
#115349=DIRECTION('ref_axis',(1.,0.,0.));
#115350=DIRECTION('center_axis',(0.,0.,-1.));
#115351=DIRECTION('ref_axis',(1.,0.,0.));
#115352=DIRECTION('center_axis',(0.,0.,1.));
#115353=DIRECTION('ref_axis',(1.,0.,0.));
#115354=DIRECTION('center_axis',(0.,0.,1.));
#115355=DIRECTION('ref_axis',(1.,0.,0.));
#115356=DIRECTION('',(0.,0.,-1.));
#115357=DIRECTION('center_axis',(0.,0.,1.));
#115358=DIRECTION('ref_axis',(1.,0.,0.));
#115359=DIRECTION('',(0.,0.,-1.));
#115360=DIRECTION('center_axis',(0.,0.,-1.));
#115361=DIRECTION('ref_axis',(1.,0.,0.));
#115362=DIRECTION('',(0.,0.,-1.));
#115363=DIRECTION('center_axis',(0.,0.,-1.));
#115364=DIRECTION('ref_axis',(1.,0.,0.));
#115365=DIRECTION('',(0.,0.,1.));
#115366=DIRECTION('center_axis',(0.,0.,1.));
#115367=DIRECTION('ref_axis',(1.,0.,0.));
#115368=DIRECTION('center_axis',(0.,0.,-1.));
#115369=DIRECTION('ref_axis',(1.,0.,0.));
#115370=DIRECTION('',(0.,0.,1.));
#115371=DIRECTION('center_axis',(0.,0.,1.));
#115372=DIRECTION('ref_axis',(1.,0.,0.));
#115373=DIRECTION('',(0.,0.,-1.));
#115374=DIRECTION('center_axis',(0.,0.,-1.));
#115375=DIRECTION('ref_axis',(1.,0.,0.));
#115376=DIRECTION('',(0.,0.,1.));
#115377=DIRECTION('center_axis',(0.,0.,1.));
#115378=DIRECTION('ref_axis',(1.,0.,0.));
#115379=DIRECTION('',(0.,0.,-1.));
#115380=DIRECTION('center_axis',(0.,0.,-1.));
#115381=DIRECTION('ref_axis',(1.,0.,0.));
#115382=DIRECTION('',(0.,0.,1.));
#115383=DIRECTION('center_axis',(0.,0.,1.));
#115384=DIRECTION('ref_axis',(1.,0.,0.));
#115385=DIRECTION('',(0.,0.,-1.));
#115386=DIRECTION('center_axis',(0.,0.,-1.));
#115387=DIRECTION('ref_axis',(1.,0.,0.));
#115388=DIRECTION('',(0.,0.,1.));
#115389=DIRECTION('center_axis',(0.,0.,1.));
#115390=DIRECTION('ref_axis',(1.,0.,0.));
#115391=DIRECTION('',(0.,0.,-1.));
#115392=DIRECTION('center_axis',(0.,0.,-1.));
#115393=DIRECTION('ref_axis',(1.,0.,0.));
#115394=DIRECTION('',(0.,0.,1.));
#115395=DIRECTION('center_axis',(0.,0.,1.));
#115396=DIRECTION('ref_axis',(1.,0.,0.));
#115397=DIRECTION('',(0.,0.,-1.));
#115398=DIRECTION('center_axis',(0.,0.,-1.));
#115399=DIRECTION('ref_axis',(1.,0.,0.));
#115400=DIRECTION('',(0.,0.,1.));
#115401=DIRECTION('center_axis',(0.,0.,1.));
#115402=DIRECTION('ref_axis',(1.,0.,0.));
#115403=DIRECTION('',(0.,0.,-1.));
#115404=DIRECTION('center_axis',(0.,0.,-1.));
#115405=DIRECTION('ref_axis',(1.,0.,0.));
#115406=DIRECTION('',(0.,0.,1.));
#115407=DIRECTION('center_axis',(0.,0.,1.));
#115408=DIRECTION('ref_axis',(1.,0.,0.));
#115409=DIRECTION('',(0.,0.,-1.));
#115410=DIRECTION('center_axis',(0.,0.,1.));
#115411=DIRECTION('ref_axis',(1.,0.,0.));
#115412=DIRECTION('center_axis',(0.,0.,-1.));
#115413=DIRECTION('ref_axis',(1.,0.,0.));
#115414=DIRECTION('center_axis',(1.22464679914735E-16,-1.,0.));
#115415=DIRECTION('ref_axis',(-1.,-1.22464679914735E-16,0.));
#115416=DIRECTION('center_axis',(0.,0.,1.));
#115417=DIRECTION('ref_axis',(1.,0.,0.));
#115418=DIRECTION('center_axis',(0.,0.,1.));
#115419=DIRECTION('ref_axis',(1.,0.,0.));
#115420=DIRECTION('center_axis',(0.,0.,-1.));
#115421=DIRECTION('ref_axis',(-1.,0.,0.));
#115422=DIRECTION('center_axis',(-1.22464679914735E-16,-1.,0.));
#115423=DIRECTION('ref_axis',(1.,-1.22464679914735E-16,0.));
#115424=DIRECTION('center_axis',(0.,0.,1.));
#115425=DIRECTION('ref_axis',(0.707106781186547,-0.707106781186548,0.));
#115426=DIRECTION('center_axis',(0.,0.,1.));
#115427=DIRECTION('ref_axis',(0.707106781186547,-0.707106781186548,0.));
#115428=DIRECTION('center_axis',(0.,0.,1.));
#115429=DIRECTION('ref_axis',(0.707106781186547,-0.707106781186548,0.));
#115430=DIRECTION('center_axis',(0.,0.,1.));
#115431=DIRECTION('ref_axis',(0.707106781186547,-0.707106781186548,0.));
#115432=DIRECTION('center_axis',(0.,0.,-1.));
#115433=DIRECTION('ref_axis',(0.707106781186547,-0.707106781186548,0.));
#115434=DIRECTION('center_axis',(0.,0.,1.));
#115435=DIRECTION('ref_axis',(0.707106781186547,-0.707106781186548,0.));
#115436=DIRECTION('center_axis',(0.,0.,-1.));
#115437=DIRECTION('ref_axis',(0.707106781186547,-0.707106781186548,0.));
#115438=DIRECTION('center_axis',(0.,0.,1.));
#115439=DIRECTION('ref_axis',(0.707106781186547,-0.707106781186548,0.));
#115440=DIRECTION('center_axis',(0.,0.,1.));
#115441=DIRECTION('ref_axis',(-1.83697019872103E-16,-1.,0.));
#115442=DIRECTION('center_axis',(0.,0.,1.));
#115443=DIRECTION('ref_axis',(-1.83697019872103E-16,-1.,0.));
#115444=DIRECTION('center_axis',(0.,0.,1.));
#115445=DIRECTION('ref_axis',(-1.83697019872103E-16,-1.,0.));
#115446=DIRECTION('center_axis',(0.,0.,1.));
#115447=DIRECTION('ref_axis',(-1.83697019872103E-16,-1.,0.));
#115448=DIRECTION('center_axis',(0.,0.,-1.));
#115449=DIRECTION('ref_axis',(-1.83697019872103E-16,-1.,0.));
#115450=DIRECTION('center_axis',(0.,0.,1.));
#115451=DIRECTION('ref_axis',(-1.83697019872103E-16,-1.,0.));
#115452=DIRECTION('center_axis',(0.,0.,-1.));
#115453=DIRECTION('ref_axis',(-1.83697019872103E-16,-1.,0.));
#115454=DIRECTION('center_axis',(0.,0.,1.));
#115455=DIRECTION('ref_axis',(-1.83697019872103E-16,-1.,0.));
#115456=DIRECTION('center_axis',(0.,0.,1.));
#115457=DIRECTION('ref_axis',(-0.707106781186548,-0.707106781186547,0.));
#115458=DIRECTION('center_axis',(0.,0.,1.));
#115459=DIRECTION('ref_axis',(-0.707106781186548,-0.707106781186548,0.));
#115460=DIRECTION('center_axis',(0.,0.,1.));
#115461=DIRECTION('ref_axis',(-0.707106781186548,-0.707106781186548,0.));
#115462=DIRECTION('center_axis',(0.,0.,1.));
#115463=DIRECTION('ref_axis',(-0.707106781186548,-0.707106781186548,0.));
#115464=DIRECTION('center_axis',(0.,0.,-1.));
#115465=DIRECTION('ref_axis',(-0.707106781186548,-0.707106781186548,0.));
#115466=DIRECTION('center_axis',(0.,0.,1.));
#115467=DIRECTION('ref_axis',(-0.707106781186548,-0.707106781186547,0.));
#115468=DIRECTION('center_axis',(0.,0.,-1.));
#115469=DIRECTION('ref_axis',(-0.707106781186548,-0.707106781186548,0.));
#115470=DIRECTION('center_axis',(0.,0.,1.));
#115471=DIRECTION('ref_axis',(-0.707106781186548,-0.707106781186548,0.));
#115472=DIRECTION('center_axis',(0.,0.,1.));
#115473=DIRECTION('ref_axis',(-1.,1.22464679914735E-16,0.));
#115474=DIRECTION('center_axis',(0.,0.,1.));
#115475=DIRECTION('ref_axis',(-1.,1.22464679914735E-16,0.));
#115476=DIRECTION('center_axis',(0.,0.,1.));
#115477=DIRECTION('ref_axis',(-1.,1.22464679914735E-16,0.));
#115478=DIRECTION('center_axis',(0.,0.,1.));
#115479=DIRECTION('ref_axis',(-1.,1.22464679914735E-16,0.));
#115480=DIRECTION('center_axis',(0.,0.,-1.));
#115481=DIRECTION('ref_axis',(-1.,1.22464679914735E-16,0.));
#115482=DIRECTION('center_axis',(0.,0.,1.));
#115483=DIRECTION('ref_axis',(-1.,1.22464679914735E-16,0.));
#115484=DIRECTION('center_axis',(0.,0.,-1.));
#115485=DIRECTION('ref_axis',(-1.,1.22464679914735E-16,0.));
#115486=DIRECTION('center_axis',(0.,0.,1.));
#115487=DIRECTION('ref_axis',(-1.,1.22464679914735E-16,0.));
#115488=DIRECTION('center_axis',(0.,0.,1.));
#115489=DIRECTION('ref_axis',(-0.707106781186547,0.707106781186548,0.));
#115490=DIRECTION('center_axis',(0.,0.,1.));
#115491=DIRECTION('ref_axis',(-0.707106781186548,0.707106781186548,0.));
#115492=DIRECTION('center_axis',(0.,0.,1.));
#115493=DIRECTION('ref_axis',(-0.707106781186548,0.707106781186548,0.));
#115494=DIRECTION('center_axis',(0.,0.,1.));
#115495=DIRECTION('ref_axis',(-0.707106781186548,0.707106781186548,0.));
#115496=DIRECTION('center_axis',(0.,0.,-1.));
#115497=DIRECTION('ref_axis',(-0.707106781186548,0.707106781186548,0.));
#115498=DIRECTION('center_axis',(0.,0.,1.));
#115499=DIRECTION('ref_axis',(-0.707106781186547,0.707106781186548,0.));
#115500=DIRECTION('center_axis',(0.,0.,-1.));
#115501=DIRECTION('ref_axis',(-0.707106781186548,0.707106781186548,0.));
#115502=DIRECTION('center_axis',(0.,0.,1.));
#115503=DIRECTION('ref_axis',(-0.707106781186548,0.707106781186548,0.));
#115504=DIRECTION('center_axis',(0.,0.,1.));
#115505=DIRECTION('ref_axis',(6.12323399573677E-17,1.,0.));
#115506=DIRECTION('center_axis',(0.,0.,1.));
#115507=DIRECTION('ref_axis',(6.12323399573677E-17,1.,0.));
#115508=DIRECTION('center_axis',(0.,0.,1.));
#115509=DIRECTION('ref_axis',(6.12323399573677E-17,1.,0.));
#115510=DIRECTION('center_axis',(0.,0.,1.));
#115511=DIRECTION('ref_axis',(6.12323399573677E-17,1.,0.));
#115512=DIRECTION('center_axis',(0.,0.,-1.));
#115513=DIRECTION('ref_axis',(6.12323399573677E-17,1.,0.));
#115514=DIRECTION('center_axis',(0.,0.,1.));
#115515=DIRECTION('ref_axis',(6.12323399573677E-17,1.,0.));
#115516=DIRECTION('center_axis',(0.,0.,-1.));
#115517=DIRECTION('ref_axis',(6.12323399573677E-17,1.,0.));
#115518=DIRECTION('center_axis',(0.,0.,1.));
#115519=DIRECTION('ref_axis',(6.12323399573677E-17,1.,0.));
#115520=DIRECTION('center_axis',(0.,0.,1.));
#115521=DIRECTION('ref_axis',(0.707106781186548,0.707106781186548,0.));
#115522=DIRECTION('center_axis',(0.,0.,1.));
#115523=DIRECTION('ref_axis',(0.707106781186548,0.707106781186548,0.));
#115524=DIRECTION('center_axis',(0.,0.,1.));
#115525=DIRECTION('ref_axis',(0.707106781186548,0.707106781186548,0.));
#115526=DIRECTION('center_axis',(0.,0.,1.));
#115527=DIRECTION('ref_axis',(0.707106781186548,0.707106781186548,0.));
#115528=DIRECTION('center_axis',(0.,0.,-1.));
#115529=DIRECTION('ref_axis',(0.707106781186548,0.707106781186548,0.));
#115530=DIRECTION('center_axis',(0.,0.,1.));
#115531=DIRECTION('ref_axis',(0.707106781186548,0.707106781186548,0.));
#115532=DIRECTION('center_axis',(0.,0.,-1.));
#115533=DIRECTION('ref_axis',(0.707106781186548,0.707106781186548,0.));
#115534=DIRECTION('center_axis',(0.,0.,1.));
#115535=DIRECTION('ref_axis',(0.707106781186548,0.707106781186548,0.));
#115536=DIRECTION('center_axis',(0.,0.,1.));
#115537=DIRECTION('ref_axis',(1.,0.,0.));
#115538=DIRECTION('center_axis',(0.,0.,1.));
#115539=DIRECTION('ref_axis',(1.,0.,0.));
#115540=DIRECTION('center_axis',(0.,0.,1.));
#115541=DIRECTION('ref_axis',(1.,0.,0.));
#115542=DIRECTION('center_axis',(0.,0.,1.));
#115543=DIRECTION('ref_axis',(1.,0.,0.));
#115544=DIRECTION('center_axis',(0.,0.,-1.));
#115545=DIRECTION('ref_axis',(1.,0.,0.));
#115546=DIRECTION('center_axis',(0.,0.,1.));
#115547=DIRECTION('ref_axis',(1.,0.,0.));
#115548=DIRECTION('center_axis',(0.,0.,-1.));
#115549=DIRECTION('ref_axis',(1.,0.,0.));
#115550=DIRECTION('center_axis',(0.,0.,1.));
#115551=DIRECTION('ref_axis',(1.,0.,0.));
#115552=DIRECTION('center_axis',(0.,0.,1.));
#115553=DIRECTION('ref_axis',(1.,0.,0.));
#115554=DIRECTION('center_axis',(0.,0.,-1.));
#115555=DIRECTION('ref_axis',(1.,0.,0.));
#115556=DIRECTION('',(0.707106781186547,8.65956056235493E-17,-0.707106781186548));
#115557=DIRECTION('center_axis',(0.,0.,1.));
#115558=DIRECTION('ref_axis',(1.,0.,0.));
#115559=DIRECTION('center_axis',(0.,0.,1.));
#115560=DIRECTION('ref_axis',(1.,0.,0.));
#115561=DIRECTION('center_axis',(0.,0.,1.));
#115562=DIRECTION('ref_axis',(1.,0.,0.));
#115563=DIRECTION('',(0.,0.,-1.));
#115564=DIRECTION('center_axis',(0.,0.,1.));
#115565=DIRECTION('ref_axis',(1.,0.,0.));
#115566=DIRECTION('center_axis',(0.,0.,-1.));
#115567=DIRECTION('ref_axis',(1.,0.,0.));
#115568=DIRECTION('',(0.707106781186547,-8.65956056235493E-17,0.707106781186548));
#115569=DIRECTION('center_axis',(0.,0.,-1.));
#115570=DIRECTION('ref_axis',(1.,0.,0.));
#115571=DIRECTION('center_axis',(0.,0.,1.));
#115572=DIRECTION('ref_axis',(1.,0.,0.));
#115573=DIRECTION('center_axis',(0.,0.,1.));
#115574=DIRECTION('ref_axis',(0.707106781186548,0.707106781186548,0.));
#115575=DIRECTION('center_axis',(0.,0.,-1.));
#115576=DIRECTION('ref_axis',(0.707106781186548,0.707106781186548,0.));
#115577=DIRECTION('',(0.500000000000022,0.500000000000022,-0.707106781186517));
#115578=DIRECTION('center_axis',(0.,0.,1.));
#115579=DIRECTION('ref_axis',(0.707106781186548,0.707106781186548,0.));
#115580=DIRECTION('center_axis',(0.,0.,1.));
#115581=DIRECTION('ref_axis',(0.707106781186548,0.707106781186548,0.));
#115582=DIRECTION('center_axis',(0.,0.,1.));
#115583=DIRECTION('ref_axis',(0.707106781186548,0.707106781186548,0.));
#115584=DIRECTION('',(0.,0.,-1.));
#115585=DIRECTION('center_axis',(0.,0.,1.));
#115586=DIRECTION('ref_axis',(0.707106781186548,0.707106781186548,0.));
#115587=DIRECTION('center_axis',(0.,0.,-1.));
#115588=DIRECTION('ref_axis',(0.707106781186548,0.707106781186548,0.));
#115589=DIRECTION('',(0.500000000000022,0.500000000000022,0.707106781186517));
#115590=DIRECTION('center_axis',(0.,0.,-1.));
#115591=DIRECTION('ref_axis',(0.707106781186548,0.707106781186548,0.));
#115592=DIRECTION('center_axis',(0.,0.,1.));
#115593=DIRECTION('ref_axis',(0.707106781186548,0.707106781186548,0.));
#115594=DIRECTION('center_axis',(0.,0.,1.));
#115595=DIRECTION('ref_axis',(6.12323399573677E-17,1.,0.));
#115596=DIRECTION('center_axis',(0.,0.,-1.));
#115597=DIRECTION('ref_axis',(6.12323399573677E-17,1.,0.));
#115598=DIRECTION('',(-4.32978028117746E-17,0.707106781186547,-0.707106781186548));
#115599=DIRECTION('center_axis',(0.,0.,1.));
#115600=DIRECTION('ref_axis',(6.12323399573677E-17,1.,0.));
#115601=DIRECTION('center_axis',(0.,0.,1.));
#115602=DIRECTION('ref_axis',(6.12323399573677E-17,1.,0.));
#115603=DIRECTION('center_axis',(0.,0.,1.));
#115604=DIRECTION('ref_axis',(6.12323399573677E-17,1.,0.));
#115605=DIRECTION('',(0.,0.,-1.));
#115606=DIRECTION('center_axis',(0.,0.,1.));
#115607=DIRECTION('ref_axis',(6.12323399573677E-17,1.,0.));
#115608=DIRECTION('center_axis',(0.,0.,-1.));
#115609=DIRECTION('ref_axis',(6.12323399573677E-17,1.,0.));
#115610=DIRECTION('',(1.29893408435324E-16,0.707106781186547,0.707106781186548));
#115611=DIRECTION('center_axis',(0.,0.,-1.));
#115612=DIRECTION('ref_axis',(6.12323399573677E-17,1.,0.));
#115613=DIRECTION('center_axis',(0.,0.,1.));
#115614=DIRECTION('ref_axis',(6.12323399573677E-17,1.,0.));
#115615=DIRECTION('center_axis',(0.,0.,1.));
#115616=DIRECTION('ref_axis',(-0.707106781186547,0.707106781186548,0.));
#115617=DIRECTION('center_axis',(0.,0.,-1.));
#115618=DIRECTION('ref_axis',(-0.707106781186547,0.707106781186548,0.));
#115619=DIRECTION('',(-0.500000000000001,0.500000000000001,-0.707106781186546));
#115620=DIRECTION('center_axis',(0.,0.,1.));
#115621=DIRECTION('ref_axis',(-0.707106781186547,0.707106781186548,0.));
#115622=DIRECTION('center_axis',(0.,0.,1.));
#115623=DIRECTION('ref_axis',(-0.707106781186547,0.707106781186548,0.));
#115624=DIRECTION('center_axis',(0.,0.,1.));
#115625=DIRECTION('ref_axis',(-0.707106781186547,0.707106781186548,0.));
#115626=DIRECTION('',(0.,0.,-1.));
#115627=DIRECTION('center_axis',(0.,0.,1.));
#115628=DIRECTION('ref_axis',(-0.707106781186547,0.707106781186548,0.));
#115629=DIRECTION('center_axis',(0.,0.,-1.));
#115630=DIRECTION('ref_axis',(-0.707106781186547,0.707106781186548,0.));
#115631=DIRECTION('',(-0.5,0.500000000000001,0.707106781186546));
#115632=DIRECTION('center_axis',(0.,0.,-1.));
#115633=DIRECTION('ref_axis',(-0.707106781186547,0.707106781186548,0.));
#115634=DIRECTION('center_axis',(0.,0.,1.));
#115635=DIRECTION('ref_axis',(-0.707106781186547,0.707106781186548,0.));
#115636=DIRECTION('center_axis',(0.,0.,1.));
#115637=DIRECTION('ref_axis',(-1.,1.22464679914735E-16,0.));
#115638=DIRECTION('center_axis',(0.,0.,-1.));
#115639=DIRECTION('ref_axis',(-1.,1.22464679914735E-16,0.));
#115640=DIRECTION('',(-0.707106781186547,-2.34655184402833E-31,-0.707106781186548));
#115641=DIRECTION('center_axis',(0.,0.,1.));
#115642=DIRECTION('ref_axis',(-1.,1.22464679914735E-16,0.));
#115643=DIRECTION('center_axis',(0.,0.,1.));
#115644=DIRECTION('ref_axis',(-1.,1.22464679914735E-16,0.));
#115645=DIRECTION('center_axis',(0.,0.,1.));
#115646=DIRECTION('ref_axis',(-1.,1.22464679914735E-16,0.));
#115647=DIRECTION('',(0.,0.,-1.));
#115648=DIRECTION('center_axis',(0.,0.,1.));
#115649=DIRECTION('ref_axis',(-1.,1.22464679914735E-16,0.));
#115650=DIRECTION('center_axis',(0.,0.,-1.));
#115651=DIRECTION('ref_axis',(-1.,1.22464679914735E-16,0.));
#115652=DIRECTION('',(-0.707106781186547,1.73191211247098E-16,0.707106781186548));
#115653=DIRECTION('center_axis',(0.,0.,-1.));
#115654=DIRECTION('ref_axis',(-1.,1.22464679914735E-16,0.));
#115655=DIRECTION('center_axis',(0.,0.,1.));
#115656=DIRECTION('ref_axis',(-1.,1.22464679914735E-16,0.));
#115657=DIRECTION('center_axis',(0.,0.,1.));
#115658=DIRECTION('ref_axis',(-0.707106781186548,-0.707106781186547,0.));
#115659=DIRECTION('center_axis',(0.,0.,-1.));
#115660=DIRECTION('ref_axis',(-0.707106781186548,-0.707106781186547,0.));
#115661=DIRECTION('',(-0.500000000000001,-0.500000000000001,-0.707106781186546));
#115662=DIRECTION('center_axis',(0.,0.,1.));
#115663=DIRECTION('ref_axis',(-0.707106781186548,-0.707106781186547,0.));
#115664=DIRECTION('center_axis',(0.,0.,1.));
#115665=DIRECTION('ref_axis',(-0.707106781186548,-0.707106781186547,0.));
#115666=DIRECTION('center_axis',(0.,0.,1.));
#115667=DIRECTION('ref_axis',(-0.707106781186548,-0.707106781186547,0.));
#115668=DIRECTION('',(0.,0.,-1.));
#115669=DIRECTION('center_axis',(0.,0.,1.));
#115670=DIRECTION('ref_axis',(-0.707106781186548,-0.707106781186547,0.));
#115671=DIRECTION('center_axis',(0.,0.,-1.));
#115672=DIRECTION('ref_axis',(-0.707106781186548,-0.707106781186547,0.));
#115673=DIRECTION('',(-0.500000000000001,-0.5,0.707106781186546));
#115674=DIRECTION('center_axis',(0.,0.,-1.));
#115675=DIRECTION('ref_axis',(-0.707106781186548,-0.707106781186547,0.));
#115676=DIRECTION('center_axis',(0.,0.,1.));
#115677=DIRECTION('ref_axis',(-0.707106781186548,-0.707106781186547,0.));
#115678=DIRECTION('center_axis',(0.,0.,1.));
#115679=DIRECTION('ref_axis',(-1.83697019872103E-16,-1.,0.));
#115680=DIRECTION('center_axis',(0.,0.,-1.));
#115681=DIRECTION('ref_axis',(-1.83697019872103E-16,-1.,0.));
#115682=DIRECTION('',(-4.32978028117747E-17,-0.707106781186547,-0.707106781186548));
#115683=DIRECTION('center_axis',(0.,0.,1.));
#115684=DIRECTION('ref_axis',(-1.83697019872103E-16,-1.,0.));
#115685=DIRECTION('center_axis',(0.,0.,1.));
#115686=DIRECTION('ref_axis',(-1.83697019872103E-16,-1.,0.));
#115687=DIRECTION('center_axis',(0.,0.,1.));
#115688=DIRECTION('ref_axis',(-1.83697019872103E-16,-1.,0.));
#115689=DIRECTION('',(0.,0.,-1.));
#115690=DIRECTION('center_axis',(0.,0.,1.));
#115691=DIRECTION('ref_axis',(-1.83697019872103E-16,-1.,0.));
#115692=DIRECTION('center_axis',(0.,0.,-1.));
#115693=DIRECTION('ref_axis',(-1.83697019872103E-16,-1.,0.));
#115694=DIRECTION('',(-2.16489014058873E-16,-0.707106781186547,0.707106781186548));
#115695=DIRECTION('center_axis',(0.,0.,-1.));
#115696=DIRECTION('ref_axis',(-1.83697019872103E-16,-1.,0.));
#115697=DIRECTION('center_axis',(0.,0.,1.));
#115698=DIRECTION('ref_axis',(-1.83697019872103E-16,-1.,0.));
#115699=DIRECTION('center_axis',(0.,0.,1.));
#115700=DIRECTION('ref_axis',(0.707106781186547,-0.707106781186548,0.));
#115701=DIRECTION('center_axis',(0.,0.,-1.));
#115702=DIRECTION('ref_axis',(0.707106781186547,-0.707106781186548,0.));
#115703=DIRECTION('',(0.500000000000001,-0.500000000000001,-0.707106781186546));
#115704=DIRECTION('center_axis',(0.,0.,1.));
#115705=DIRECTION('ref_axis',(0.707106781186547,-0.707106781186548,0.));
#115706=DIRECTION('center_axis',(0.,0.,1.));
#115707=DIRECTION('ref_axis',(0.707106781186547,-0.707106781186548,0.));
#115708=DIRECTION('center_axis',(0.,0.,1.));
#115709=DIRECTION('ref_axis',(0.707106781186547,-0.707106781186548,0.));
#115710=DIRECTION('',(0.,0.,-1.));
#115711=DIRECTION('center_axis',(0.,0.,1.));
#115712=DIRECTION('ref_axis',(0.707106781186547,-0.707106781186548,0.));
#115713=DIRECTION('center_axis',(0.,0.,-1.));
#115714=DIRECTION('ref_axis',(0.707106781186547,-0.707106781186548,0.));
#115715=DIRECTION('',(0.5,-0.500000000000001,0.707106781186546));
#115716=DIRECTION('center_axis',(0.,0.,-1.));
#115717=DIRECTION('ref_axis',(0.707106781186547,-0.707106781186548,0.));
#115718=DIRECTION('center_axis',(0.,0.,1.));
#115719=DIRECTION('ref_axis',(0.707106781186547,-0.707106781186548,0.));
#358160=CARTESIAN_POINT('',(0.,0.,0.));
#358161=CARTESIAN_POINT('Origin',(0.,0.,-3.33333333333333));
#358162=CARTESIAN_POINT('',(-1.76666666666667,2.16354267849366E-16,-3.5));
#358163=CARTESIAN_POINT('Origin',(0.,0.,-3.5));
#358164=CARTESIAN_POINT('',(-1.6,-1.95943487863577E-16,-3.33333333333333));
#358165=CARTESIAN_POINT('Origin',(-1.76666666666667,-2.16354267849366E-16,
-3.33333333333333));
#358166=CARTESIAN_POINT('Origin',(0.,0.,-3.33333333333333));
#358167=CARTESIAN_POINT('Origin',(0.,0.,-3.5));
#358168=CARTESIAN_POINT('',(2.23333333333333,-2.73504451809576E-16,-3.5));
#358169=CARTESIAN_POINT('Origin',(0.,0.,-3.5));
#358170=CARTESIAN_POINT('Origin',(0.,0.,0.));
#358171=CARTESIAN_POINT('',(-1.6,-1.95943487863577E-16,-3.));
#358172=CARTESIAN_POINT('',(-1.6,-1.95943487863577E-16,0.));
#358173=CARTESIAN_POINT('',(-1.57109375,-0.302761339524943,-3.));
#358174=CARTESIAN_POINT('Origin',(0.,0.,-3.));
#358175=CARTESIAN_POINT('',(-1.57109375,-0.302761339524943,3.));
#358176=CARTESIAN_POINT('',(-1.57109375,-0.302761339524943,0.));
#358177=CARTESIAN_POINT('',(-1.6,-1.95943487863577E-16,3.));
#358178=CARTESIAN_POINT('Origin',(0.,0.,3.));
#358179=CARTESIAN_POINT('',(-1.6,-1.95943487863577E-16,3.33333333333333));
#358180=CARTESIAN_POINT('',(-1.6,-1.95943487863577E-16,0.));
#358181=CARTESIAN_POINT('',(1.6,-1.95943487863577E-16,3.33333333333333));
#358182=CARTESIAN_POINT('Origin',(0.,0.,3.33333333333333));
#358183=CARTESIAN_POINT('Origin',(0.,0.,3.33333333333333));
#358184=CARTESIAN_POINT('',(-1.57109375,0.302761339524943,3.));
#358185=CARTESIAN_POINT('Origin',(0.,0.,3.));
#358186=CARTESIAN_POINT('',(-1.57109375,0.302761339524943,-3.));
#358187=CARTESIAN_POINT('',(-1.57109375,0.302761339524943,0.));
#358188=CARTESIAN_POINT('Origin',(0.,0.,-3.));
#358189=CARTESIAN_POINT('',(0.896846448245593,-1.32501564076401,-3.));
#358190=CARTESIAN_POINT('',(1.32501564076401,-0.896846448245593,-3.));
#358191=CARTESIAN_POINT('Origin',(0.,0.,-3.));
#358192=CARTESIAN_POINT('',(1.32501564076401,-0.896846448245593,3.));
#358193=CARTESIAN_POINT('',(1.32501564076401,-0.896846448245593,0.));
#358194=CARTESIAN_POINT('',(0.896846448245593,-1.32501564076401,3.));
#358195=CARTESIAN_POINT('Origin',(0.,0.,3.));
#358196=CARTESIAN_POINT('',(0.896846448245593,-1.32501564076401,0.));
#358197=CARTESIAN_POINT('',(-0.302761339524943,-1.57109375,-3.));
#358198=CARTESIAN_POINT('',(0.302761339524943,-1.57109375,-3.));
#358199=CARTESIAN_POINT('Origin',(0.,0.,-3.));
#358200=CARTESIAN_POINT('',(0.302761339524943,-1.57109375,3.));
#358201=CARTESIAN_POINT('',(0.302761339524943,-1.57109375,0.));
#358202=CARTESIAN_POINT('',(-0.302761339524943,-1.57109375,3.));
#358203=CARTESIAN_POINT('Origin',(0.,0.,3.));
#358204=CARTESIAN_POINT('',(-0.302761339524943,-1.57109375,0.));
#358205=CARTESIAN_POINT('',(-1.32501564076401,-0.896846448245593,-3.));
#358206=CARTESIAN_POINT('',(-0.896846448245593,-1.32501564076401,-3.));
#358207=CARTESIAN_POINT('Origin',(0.,0.,-3.));
#358208=CARTESIAN_POINT('',(-0.896846448245593,-1.32501564076401,3.));
#358209=CARTESIAN_POINT('',(-0.896846448245593,-1.32501564076401,0.));
#358210=CARTESIAN_POINT('',(-1.32501564076401,-0.896846448245593,3.));
#358211=CARTESIAN_POINT('Origin',(0.,0.,3.));
#358212=CARTESIAN_POINT('',(-1.32501564076401,-0.896846448245593,0.));
#358213=CARTESIAN_POINT('',(-0.896846448245593,1.32501564076401,-3.));
#358214=CARTESIAN_POINT('',(-1.32501564076401,0.896846448245593,-3.));
#358215=CARTESIAN_POINT('Origin',(0.,0.,-3.));
#358216=CARTESIAN_POINT('',(-1.32501564076401,0.896846448245593,3.));
#358217=CARTESIAN_POINT('',(-1.32501564076401,0.896846448245593,0.));
#358218=CARTESIAN_POINT('',(-0.896846448245593,1.32501564076401,3.));
#358219=CARTESIAN_POINT('Origin',(0.,0.,3.));
#358220=CARTESIAN_POINT('',(-0.896846448245593,1.32501564076401,0.));
#358221=CARTESIAN_POINT('',(0.302761339524943,1.57109375,-3.));
#358222=CARTESIAN_POINT('',(-0.302761339524943,1.57109375,-3.));
#358223=CARTESIAN_POINT('Origin',(0.,0.,-3.));
#358224=CARTESIAN_POINT('',(-0.302761339524943,1.57109375,3.));
#358225=CARTESIAN_POINT('',(-0.302761339524943,1.57109375,0.));
#358226=CARTESIAN_POINT('',(0.302761339524943,1.57109375,3.));
#358227=CARTESIAN_POINT('Origin',(0.,0.,3.));
#358228=CARTESIAN_POINT('',(0.302761339524943,1.57109375,0.));
#358229=CARTESIAN_POINT('',(1.32501564076401,0.896846448245593,-3.));
#358230=CARTESIAN_POINT('',(0.896846448245593,1.32501564076401,-3.));
#358231=CARTESIAN_POINT('Origin',(0.,0.,-3.));
#358232=CARTESIAN_POINT('',(0.896846448245593,1.32501564076401,3.));
#358233=CARTESIAN_POINT('',(0.896846448245593,1.32501564076401,0.));
#358234=CARTESIAN_POINT('',(1.32501564076401,0.896846448245593,3.));
#358235=CARTESIAN_POINT('Origin',(0.,0.,3.));
#358236=CARTESIAN_POINT('',(1.32501564076401,0.896846448245593,0.));
#358237=CARTESIAN_POINT('',(1.57109375,-0.302761339524943,-3.));
#358238=CARTESIAN_POINT('',(1.57109375,0.302761339524943,-3.));
#358239=CARTESIAN_POINT('Origin',(0.,0.,-3.));
#358240=CARTESIAN_POINT('',(1.57109375,0.302761339524943,3.));
#358241=CARTESIAN_POINT('',(1.57109375,0.302761339524943,0.));
#358242=CARTESIAN_POINT('',(1.57109375,-0.302761339524943,3.));
#358243=CARTESIAN_POINT('Origin',(0.,0.,3.));
#358244=CARTESIAN_POINT('',(1.57109375,-0.302761339524943,0.));
#358245=CARTESIAN_POINT('Origin',(0.,0.,-3.33333333333333));
#358246=CARTESIAN_POINT('',(2.4,-2.93915231795365E-16,-3.33333333333333));
#358247=CARTESIAN_POINT('Origin',(2.23333333333333,-2.73504451809575E-16,
-3.33333333333333));
#358248=CARTESIAN_POINT('',(-2.4,2.93915231795365E-16,-3.33333333333333));
#358249=CARTESIAN_POINT('Origin',(0.,0.,-3.33333333333333));
#358250=CARTESIAN_POINT('Origin',(0.,0.,-3.33333333333333));
#358251=CARTESIAN_POINT('Origin',(0.,0.,0.));
#358252=CARTESIAN_POINT('',(-2.4,-2.93915231795365E-16,3.33333333333333));
#358253=CARTESIAN_POINT('Origin',(0.,0.,3.33333333333333));
#358254=CARTESIAN_POINT('',(-2.4,-2.93915231795365E-16,3.));
#358255=CARTESIAN_POINT('',(-2.4,-2.93915231795365E-16,0.));
#358256=CARTESIAN_POINT('',(-2.37109375,-0.371368319476685,3.));
#358257=CARTESIAN_POINT('Origin',(0.,0.,3.));
#358258=CARTESIAN_POINT('',(-2.37109375,-0.371368319476685,-3.));
#358259=CARTESIAN_POINT('',(-2.37109375,-0.371368319476685,0.));
#358260=CARTESIAN_POINT('',(-2.4,-2.93915231795365E-16,-3.));
#358261=CARTESIAN_POINT('Origin',(0.,0.,-3.));
#358262=CARTESIAN_POINT('',(-2.4,-2.93915231795365E-16,0.));
#358263=CARTESIAN_POINT('',(-2.37109375,0.371368319476686,-3.));
#358264=CARTESIAN_POINT('Origin',(0.,0.,-3.));
#358265=CARTESIAN_POINT('',(-2.37109375,0.371368319476686,3.));
#358266=CARTESIAN_POINT('',(-2.37109375,0.371368319476686,0.));
#358267=CARTESIAN_POINT('Origin',(0.,0.,3.));
#358268=CARTESIAN_POINT('',(1.93921352647386,-1.41401941243422,-3.));
#358269=CARTESIAN_POINT('',(1.41401941243422,-1.93921352647386,-3.));
#358270=CARTESIAN_POINT('Origin',(0.,0.,-3.));
#358271=CARTESIAN_POINT('',(1.41401941243422,-1.93921352647386,3.));
#358272=CARTESIAN_POINT('',(1.41401941243422,-1.93921352647386,0.));
#358273=CARTESIAN_POINT('',(1.93921352647386,-1.41401941243422,3.));
#358274=CARTESIAN_POINT('Origin',(0.,0.,3.));
#358275=CARTESIAN_POINT('',(1.93921352647386,-1.41401941243422,0.));
#358276=CARTESIAN_POINT('',(0.371368319476685,-2.37109375,-3.));
#358277=CARTESIAN_POINT('',(-0.371368319476686,-2.37109375,-3.));
#358278=CARTESIAN_POINT('Origin',(0.,0.,-3.));
#358279=CARTESIAN_POINT('',(-0.371368319476686,-2.37109375,3.));
#358280=CARTESIAN_POINT('',(-0.371368319476686,-2.37109375,0.));
#358281=CARTESIAN_POINT('',(0.371368319476685,-2.37109375,3.));
#358282=CARTESIAN_POINT('Origin',(0.,0.,3.));
#358283=CARTESIAN_POINT('',(0.371368319476685,-2.37109375,0.));
#358284=CARTESIAN_POINT('',(-1.41401941243422,-1.93921352647386,-3.));
#358285=CARTESIAN_POINT('',(-1.93921352647386,-1.41401941243422,-3.));
#358286=CARTESIAN_POINT('Origin',(0.,0.,-3.));
#358287=CARTESIAN_POINT('',(-1.93921352647386,-1.41401941243422,3.));
#358288=CARTESIAN_POINT('',(-1.93921352647386,-1.41401941243422,0.));
#358289=CARTESIAN_POINT('',(-1.41401941243422,-1.93921352647386,3.));
#358290=CARTESIAN_POINT('Origin',(0.,0.,3.));
#358291=CARTESIAN_POINT('',(-1.41401941243422,-1.93921352647386,0.));
#358292=CARTESIAN_POINT('',(-1.93921352647386,1.41401941243422,-3.));
#358293=CARTESIAN_POINT('',(-1.41401941243422,1.93921352647386,-3.));
#358294=CARTESIAN_POINT('Origin',(0.,0.,-3.));
#358295=CARTESIAN_POINT('',(-1.41401941243422,1.93921352647386,3.));
#358296=CARTESIAN_POINT('',(-1.41401941243422,1.93921352647386,0.));
#358297=CARTESIAN_POINT('',(-1.93921352647386,1.41401941243422,3.));
#358298=CARTESIAN_POINT('Origin',(0.,0.,3.));
#358299=CARTESIAN_POINT('',(-1.93921352647386,1.41401941243422,0.));
#358300=CARTESIAN_POINT('',(-0.371368319476685,2.37109375,-3.));
#358301=CARTESIAN_POINT('',(0.371368319476686,2.37109375,-3.));
#358302=CARTESIAN_POINT('Origin',(0.,0.,-3.));
#358303=CARTESIAN_POINT('',(0.371368319476686,2.37109375,3.));
#358304=CARTESIAN_POINT('',(0.371368319476686,2.37109375,0.));
#358305=CARTESIAN_POINT('',(-0.371368319476685,2.37109375,3.));
#358306=CARTESIAN_POINT('Origin',(0.,0.,3.));
#358307=CARTESIAN_POINT('',(-0.371368319476685,2.37109375,0.));
#358308=CARTESIAN_POINT('',(1.41401941243422,1.93921352647386,-3.));
#358309=CARTESIAN_POINT('',(1.93921352647386,1.41401941243422,-3.));
#358310=CARTESIAN_POINT('Origin',(0.,0.,-3.));
#358311=CARTESIAN_POINT('',(1.93921352647386,1.41401941243422,3.));
#358312=CARTESIAN_POINT('',(1.93921352647386,1.41401941243422,0.));
#358313=CARTESIAN_POINT('',(1.41401941243422,1.93921352647386,3.));
#358314=CARTESIAN_POINT('Origin',(0.,0.,3.));
#358315=CARTESIAN_POINT('',(1.41401941243422,1.93921352647386,0.));
#358316=CARTESIAN_POINT('',(2.37109375,0.371368319476686,-3.));
#358317=CARTESIAN_POINT('',(2.37109375,-0.371368319476686,-3.));
#358318=CARTESIAN_POINT('Origin',(0.,0.,-3.));
#358319=CARTESIAN_POINT('',(2.37109375,-0.371368319476686,3.));
#358320=CARTESIAN_POINT('',(2.37109375,-0.371368319476686,0.));
#358321=CARTESIAN_POINT('',(2.37109375,0.371368319476686,3.));
#358322=CARTESIAN_POINT('Origin',(0.,0.,3.));
#358323=CARTESIAN_POINT('',(2.37109375,0.371368319476686,0.));
#358324=CARTESIAN_POINT('Origin',(0.,0.,3.33333333333333));
#358325=CARTESIAN_POINT('',(-2.23333333333333,2.73504451809576E-16,3.5));
#358326=CARTESIAN_POINT('Origin',(0.,0.,3.5));
#358327=CARTESIAN_POINT('Origin',(-2.23333333333333,-2.73504451809575E-16,
3.33333333333333));
#358328=CARTESIAN_POINT('Origin',(0.,0.,3.5));
#358329=CARTESIAN_POINT('',(1.76666666666667,-2.16354267849366E-16,3.5));
#358330=CARTESIAN_POINT('Origin',(0.,0.,3.5));
#358331=CARTESIAN_POINT('Origin',(0.,0.,3.33333333333333));
#358332=CARTESIAN_POINT('Origin',(1.76666666666667,-2.16354267849366E-16,
3.33333333333333));
#358333=CARTESIAN_POINT('Origin',(1.41421356237309,-1.4142135623731,3.));
#358334=CARTESIAN_POINT('Origin',(1.41421356237309,-1.4142135623731,3.));
#358335=CARTESIAN_POINT('Origin',(1.41421356237309,-1.4142135623731,3.));
#358336=CARTESIAN_POINT('Origin',(1.41421356237309,-1.4142135623731,0.));
#358337=CARTESIAN_POINT('Origin',(1.41421356237309,-1.4142135623731,-3.));
#358338=CARTESIAN_POINT('Origin',(1.41421356237309,-1.4142135623731,-3.));
#358339=CARTESIAN_POINT('Origin',(1.41421356237309,-1.4142135623731,-3.));
#358340=CARTESIAN_POINT('Origin',(1.41421356237309,-1.4142135623731,0.));
#358341=CARTESIAN_POINT('Origin',(-3.67394039744206E-16,-2.,3.));
#358342=CARTESIAN_POINT('Origin',(-3.67394039744206E-16,-2.,3.));
#358343=CARTESIAN_POINT('Origin',(-3.67394039744206E-16,-2.,3.));
#358344=CARTESIAN_POINT('Origin',(-3.67394039744206E-16,-2.,0.));
#358345=CARTESIAN_POINT('Origin',(-3.67394039744206E-16,-2.,-3.));
#358346=CARTESIAN_POINT('Origin',(-3.67394039744206E-16,-2.,-3.));
#358347=CARTESIAN_POINT('Origin',(-3.67394039744206E-16,-2.,-3.));
#358348=CARTESIAN_POINT('Origin',(-3.67394039744206E-16,-2.,0.));
#358349=CARTESIAN_POINT('Origin',(-1.4142135623731,-1.41421356237309,3.));
#358350=CARTESIAN_POINT('Origin',(-1.4142135623731,-1.41421356237309,3.));
#358351=CARTESIAN_POINT('Origin',(-1.4142135623731,-1.41421356237309,3.));
#358352=CARTESIAN_POINT('Origin',(-1.4142135623731,-1.41421356237309,0.));
#358353=CARTESIAN_POINT('Origin',(-1.4142135623731,-1.41421356237309,-3.));
#358354=CARTESIAN_POINT('Origin',(-1.4142135623731,-1.41421356237309,-3.));
#358355=CARTESIAN_POINT('Origin',(-1.4142135623731,-1.41421356237309,-3.));
#358356=CARTESIAN_POINT('Origin',(-1.4142135623731,-1.41421356237309,0.));
#358357=CARTESIAN_POINT('Origin',(-2.,2.44929359829471E-16,3.));
#358358=CARTESIAN_POINT('Origin',(-2.,2.44929359829471E-16,3.));
#358359=CARTESIAN_POINT('Origin',(-2.,2.44929359829471E-16,3.));
#358360=CARTESIAN_POINT('Origin',(-2.,2.44929359829471E-16,0.));
#358361=CARTESIAN_POINT('Origin',(-2.,2.44929359829471E-16,-3.));
#358362=CARTESIAN_POINT('Origin',(-2.,2.44929359829471E-16,-3.));
#358363=CARTESIAN_POINT('Origin',(-2.,2.44929359829471E-16,-3.));
#358364=CARTESIAN_POINT('Origin',(-2.,2.44929359829471E-16,0.));
#358365=CARTESIAN_POINT('Origin',(-1.41421356237309,1.4142135623731,3.));
#358366=CARTESIAN_POINT('Origin',(-1.41421356237309,1.4142135623731,3.));
#358367=CARTESIAN_POINT('Origin',(-1.41421356237309,1.4142135623731,3.));
#358368=CARTESIAN_POINT('Origin',(-1.41421356237309,1.4142135623731,0.));
#358369=CARTESIAN_POINT('Origin',(-1.41421356237309,1.4142135623731,-3.));
#358370=CARTESIAN_POINT('Origin',(-1.41421356237309,1.4142135623731,-3.));
#358371=CARTESIAN_POINT('Origin',(-1.41421356237309,1.4142135623731,-3.));
#358372=CARTESIAN_POINT('Origin',(-1.41421356237309,1.4142135623731,0.));
#358373=CARTESIAN_POINT('Origin',(1.22464679914735E-16,2.,3.));
#358374=CARTESIAN_POINT('Origin',(1.22464679914735E-16,2.,3.));
#358375=CARTESIAN_POINT('Origin',(1.22464679914735E-16,2.,3.));
#358376=CARTESIAN_POINT('Origin',(1.22464679914735E-16,2.,0.));
#358377=CARTESIAN_POINT('Origin',(1.22464679914735E-16,2.,-3.));
#358378=CARTESIAN_POINT('Origin',(1.22464679914735E-16,2.,-3.));
#358379=CARTESIAN_POINT('Origin',(1.22464679914735E-16,2.,-3.));
#358380=CARTESIAN_POINT('Origin',(1.22464679914735E-16,2.,0.));
#358381=CARTESIAN_POINT('Origin',(1.4142135623731,1.4142135623731,3.));
#358382=CARTESIAN_POINT('Origin',(1.4142135623731,1.4142135623731,3.));
#358383=CARTESIAN_POINT('Origin',(1.4142135623731,1.4142135623731,3.));
#358384=CARTESIAN_POINT('Origin',(1.4142135623731,1.4142135623731,0.));
#358385=CARTESIAN_POINT('Origin',(1.4142135623731,1.4142135623731,-3.));
#358386=CARTESIAN_POINT('Origin',(1.4142135623731,1.4142135623731,-3.));
#358387=CARTESIAN_POINT('Origin',(1.4142135623731,1.4142135623731,-3.));
#358388=CARTESIAN_POINT('Origin',(1.4142135623731,1.4142135623731,0.));
#358389=CARTESIAN_POINT('Origin',(2.,0.,3.));
#358390=CARTESIAN_POINT('Origin',(2.,0.,3.));
#358391=CARTESIAN_POINT('Origin',(2.,0.,3.));
#358392=CARTESIAN_POINT('Origin',(2.,0.,0.));
#358393=CARTESIAN_POINT('Origin',(2.,0.,-3.));
#358394=CARTESIAN_POINT('Origin',(2.,0.,-3.));
#358395=CARTESIAN_POINT('Origin',(2.,0.,-3.));
#358396=CARTESIAN_POINT('Origin',(2.,0.,0.));
#358397=CARTESIAN_POINT('Origin',(2.,0.,-2.9625));
#358398=CARTESIAN_POINT('',(1.5,6.12323399573676E-17,-2.95));
#358399=CARTESIAN_POINT('Origin',(2.,0.,-2.95));
#358400=CARTESIAN_POINT('',(1.525,-5.81707229594993E-17,-2.975));
#358401=CARTESIAN_POINT('',(1.5125,-5.97015314584335E-17,-2.9625));
#358402=CARTESIAN_POINT('Origin',(2.,0.,-2.975));
#358403=CARTESIAN_POINT('Origin',(2.,0.,0.));
#358404=CARTESIAN_POINT('',(1.5,-6.12323399573676E-17,2.95));
#358405=CARTESIAN_POINT('Origin',(2.,0.,2.95));
#358406=CARTESIAN_POINT('',(1.5,-6.12323399573677E-17,0.));
#358407=CARTESIAN_POINT('Origin',(2.,0.,-2.975));
#358408=CARTESIAN_POINT('Origin',(2.,0.,2.9625));
#358409=CARTESIAN_POINT('',(1.525,5.81707229594993E-17,2.975));
#358410=CARTESIAN_POINT('',(1.5125,5.97015314584335E-17,2.9625));
#358411=CARTESIAN_POINT('Origin',(2.,0.,2.975));
#358412=CARTESIAN_POINT('Origin',(2.,0.,2.975));
#358413=CARTESIAN_POINT('Origin',(1.4142135623731,1.4142135623731,-2.9625));
#358414=CARTESIAN_POINT('',(1.06066017177982,1.06066017177982,-2.95));
#358415=CARTESIAN_POINT('Origin',(1.4142135623731,1.4142135623731,-2.95));
#358416=CARTESIAN_POINT('',(1.07833784130949,1.07833784130949,-2.975));
#358417=CARTESIAN_POINT('',(1.06949900654466,1.06949900654466,-2.9625));
#358418=CARTESIAN_POINT('Origin',(1.4142135623731,1.4142135623731,-2.975));
#358419=CARTESIAN_POINT('Origin',(1.4142135623731,1.4142135623731,0.));
#358420=CARTESIAN_POINT('',(1.06066017177982,1.06066017177982,2.95));
#358421=CARTESIAN_POINT('Origin',(1.4142135623731,1.4142135623731,2.95));
#358422=CARTESIAN_POINT('',(1.06066017177983,1.06066017177983,0.));
#358423=CARTESIAN_POINT('Origin',(1.4142135623731,1.4142135623731,-2.975));
#358424=CARTESIAN_POINT('Origin',(1.4142135623731,1.4142135623731,2.9625));
#358425=CARTESIAN_POINT('',(1.07833784130949,1.07833784130949,2.975));
#358426=CARTESIAN_POINT('',(1.06949900654466,1.06949900654466,2.9625));
#358427=CARTESIAN_POINT('Origin',(1.4142135623731,1.4142135623731,2.975));
#358428=CARTESIAN_POINT('Origin',(1.4142135623731,1.4142135623731,2.975));
#358429=CARTESIAN_POINT('Origin',(1.22464679914735E-16,2.,-2.9625));
#358430=CARTESIAN_POINT('',(3.06161699786839E-17,1.5,-2.95));
#358431=CARTESIAN_POINT('Origin',(1.22464679914735E-16,2.,-2.95));
#358432=CARTESIAN_POINT('',(1.51550041394485E-16,1.525,-2.975));
#358433=CARTESIAN_POINT('',(1.52315445643952E-16,1.5125,-2.9625));
#358434=CARTESIAN_POINT('Origin',(1.22464679914735E-16,2.,-2.975));
#358435=CARTESIAN_POINT('Origin',(1.22464679914735E-16,2.,0.));
#358436=CARTESIAN_POINT('',(1.53080849893419E-16,1.5,2.95));
#358437=CARTESIAN_POINT('Origin',(1.22464679914735E-16,2.,2.95));
#358438=CARTESIAN_POINT('',(1.53080849893419E-16,1.5,0.));
#358439=CARTESIAN_POINT('Origin',(1.22464679914735E-16,2.,-2.975));
#358440=CARTESIAN_POINT('Origin',(1.22464679914735E-16,2.,2.9625));
#358441=CARTESIAN_POINT('',(3.52085954754864E-17,1.525,2.975));
#358442=CARTESIAN_POINT('',(3.29123827270848E-17,1.5125,2.9625));
#358443=CARTESIAN_POINT('Origin',(1.22464679914735E-16,2.,2.975));
#358444=CARTESIAN_POINT('Origin',(1.22464679914735E-16,2.,2.975));
#358445=CARTESIAN_POINT('Origin',(-1.41421356237309,1.4142135623731,-2.9625));
#358446=CARTESIAN_POINT('',(-1.06066017177982,1.06066017177982,-2.95));
#358447=CARTESIAN_POINT('Origin',(-1.41421356237309,1.4142135623731,-2.95));
#358448=CARTESIAN_POINT('',(-1.07833784130949,1.07833784130949,-2.975));
#358449=CARTESIAN_POINT('',(-1.06949900654465,1.06949900654466,-2.9625));
#358450=CARTESIAN_POINT('Origin',(-1.41421356237309,1.4142135623731,-2.975));
#358451=CARTESIAN_POINT('Origin',(-1.41421356237309,1.4142135623731,0.));
#358452=CARTESIAN_POINT('',(-1.06066017177982,1.06066017177982,2.95));
#358453=CARTESIAN_POINT('Origin',(-1.41421356237309,1.4142135623731,2.95));
#358454=CARTESIAN_POINT('',(-1.06066017177982,1.06066017177983,0.));
#358455=CARTESIAN_POINT('Origin',(-1.41421356237309,1.4142135623731,-2.975));
#358456=CARTESIAN_POINT('Origin',(-1.41421356237309,1.4142135623731,2.9625));
#358457=CARTESIAN_POINT('',(-1.07833784130949,1.07833784130949,2.975));
#358458=CARTESIAN_POINT('',(-1.06949900654465,1.06949900654466,2.9625));
#358459=CARTESIAN_POINT('Origin',(-1.41421356237309,1.4142135623731,2.975));
#358460=CARTESIAN_POINT('Origin',(-1.41421356237309,1.4142135623731,2.975));
#358461=CARTESIAN_POINT('Origin',(-2.,2.44929359829471E-16,-2.9625));
#358462=CARTESIAN_POINT('',(-1.5,1.22464679914735E-16,-2.95));
#358463=CARTESIAN_POINT('Origin',(-2.,2.44929359829471E-16,-2.95));
#358464=CARTESIAN_POINT('',(-1.525,2.44929359829471E-16,-2.975));
#358465=CARTESIAN_POINT('',(-1.5125,2.44929359829471E-16,-2.9625));
#358466=CARTESIAN_POINT('Origin',(-2.,2.44929359829471E-16,-2.975));
#358467=CARTESIAN_POINT('Origin',(-2.,2.44929359829471E-16,0.));
#358468=CARTESIAN_POINT('',(-1.5,2.44929359829471E-16,2.95));
#358469=CARTESIAN_POINT('Origin',(-2.,2.44929359829471E-16,2.95));
#358470=CARTESIAN_POINT('',(-1.5,2.44929359829471E-16,0.));
#358471=CARTESIAN_POINT('Origin',(-2.,2.44929359829471E-16,-2.975));
#358472=CARTESIAN_POINT('Origin',(-2.,2.44929359829471E-16,2.9625));
#358473=CARTESIAN_POINT('',(-1.525,1.28587913910472E-16,2.975));
#358474=CARTESIAN_POINT('',(-1.5125,1.25526296912604E-16,2.9625));
#358475=CARTESIAN_POINT('Origin',(-2.,2.44929359829471E-16,2.975));
#358476=CARTESIAN_POINT('Origin',(-2.,2.44929359829471E-16,2.975));
#358477=CARTESIAN_POINT('Origin',(-1.4142135623731,-1.41421356237309,-2.9625));
#358478=CARTESIAN_POINT('',(-1.06066017177982,-1.06066017177982,-2.95));
#358479=CARTESIAN_POINT('Origin',(-1.4142135623731,-1.41421356237309,-2.95));
#358480=CARTESIAN_POINT('',(-1.07833784130949,-1.07833784130949,-2.975));
#358481=CARTESIAN_POINT('',(-1.06949900654466,-1.06949900654465,-2.9625));
#358482=CARTESIAN_POINT('Origin',(-1.4142135623731,-1.41421356237309,-2.975));
#358483=CARTESIAN_POINT('Origin',(-1.4142135623731,-1.41421356237309,0.));
#358484=CARTESIAN_POINT('',(-1.06066017177982,-1.06066017177982,2.95));
#358485=CARTESIAN_POINT('Origin',(-1.4142135623731,-1.41421356237309,2.95));
#358486=CARTESIAN_POINT('',(-1.06066017177983,-1.06066017177982,0.));
#358487=CARTESIAN_POINT('Origin',(-1.4142135623731,-1.41421356237309,-2.975));
#358488=CARTESIAN_POINT('Origin',(-1.4142135623731,-1.41421356237309,2.9625));
#358489=CARTESIAN_POINT('',(-1.07833784130949,-1.07833784130949,2.975));
#358490=CARTESIAN_POINT('',(-1.06949900654466,-1.06949900654465,2.9625));
#358491=CARTESIAN_POINT('Origin',(-1.4142135623731,-1.41421356237309,2.975));
#358492=CARTESIAN_POINT('Origin',(-1.4142135623731,-1.41421356237309,2.975));
#358493=CARTESIAN_POINT('Origin',(-3.67394039744206E-16,-2.,-2.9625));
#358494=CARTESIAN_POINT('',(-2.14313189850787E-16,-1.5,-2.95));
#358495=CARTESIAN_POINT('Origin',(-3.67394039744206E-16,-2.,-2.95));
#358496=CARTESIAN_POINT('',(-3.38308678264456E-16,-1.525,-2.975));
#358497=CARTESIAN_POINT('',(-3.37543274014989E-16,-1.5125,-2.9625));
#358498=CARTESIAN_POINT('Origin',(-3.67394039744206E-16,-2.,-2.975));
#358499=CARTESIAN_POINT('Origin',(-3.67394039744206E-16,-2.,0.));
#358500=CARTESIAN_POINT('',(-3.36777869765522E-16,-1.5,2.95));
#358501=CARTESIAN_POINT('Origin',(-3.67394039744206E-16,-2.,2.95));
#358502=CARTESIAN_POINT('',(-3.36777869765522E-16,-1.5,0.));
#358503=CARTESIAN_POINT('Origin',(-3.67394039744206E-16,-2.,-2.975));
#358504=CARTESIAN_POINT('Origin',(-3.67394039744206E-16,-2.,2.9625));
#358505=CARTESIAN_POINT('',(-2.21967232345458E-16,-1.525,2.975));
#358506=CARTESIAN_POINT('',(-2.18140211098122E-16,-1.5125,2.9625));
#358507=CARTESIAN_POINT('Origin',(-3.67394039744206E-16,-2.,2.975));
#358508=CARTESIAN_POINT('Origin',(-3.67394039744206E-16,-2.,2.975));
#358509=CARTESIAN_POINT('Origin',(1.41421356237309,-1.4142135623731,-2.9625));
#358510=CARTESIAN_POINT('',(1.06066017177982,-1.06066017177982,-2.95));
#358511=CARTESIAN_POINT('Origin',(1.41421356237309,-1.4142135623731,-2.95));
#358512=CARTESIAN_POINT('',(1.07833784130948,-1.07833784130949,-2.975));
#358513=CARTESIAN_POINT('',(1.06949900654465,-1.06949900654466,-2.9625));
#358514=CARTESIAN_POINT('Origin',(1.41421356237309,-1.4142135623731,-2.975));
#358515=CARTESIAN_POINT('Origin',(1.41421356237309,-1.4142135623731,0.));
#358516=CARTESIAN_POINT('',(1.06066017177982,-1.06066017177982,2.95));
#358517=CARTESIAN_POINT('Origin',(1.41421356237309,-1.4142135623731,2.95));
#358518=CARTESIAN_POINT('',(1.06066017177982,-1.06066017177983,0.));
#358519=CARTESIAN_POINT('Origin',(1.41421356237309,-1.4142135623731,-2.975));
#358520=CARTESIAN_POINT('Origin',(1.41421356237309,-1.4142135623731,2.9625));
#358521=CARTESIAN_POINT('',(1.07833784130948,-1.07833784130949,2.975));
#358522=CARTESIAN_POINT('',(1.06949900654465,-1.06949900654466,2.9625));
#358523=CARTESIAN_POINT('Origin',(1.41421356237309,-1.4142135623731,2.975));
#358524=CARTESIAN_POINT('Origin',(1.41421356237309,-1.4142135623731,2.975));
#459201=UNCERTAINTY_MEASURE_WITH_UNIT(LENGTH_MEASURE(0.01),#459243,
'DISTANCE_ACCURACY_VALUE',
'Maximum model space distance between geometric entities at asserted c
onnectivities');
#459216=UNCERTAINTY_MEASURE_WITH_UNIT(LENGTH_MEASURE(0.01),#459243,
'DISTANCE_ACCURACY_VALUE',
'Maximum model space distance between geometric entities at asserted c
onnectivities');
#459227=(
GEOMETRIC_REPRESENTATION_CONTEXT(3)
GLOBAL_UNCERTAINTY_ASSIGNED_CONTEXT((#459201))
GLOBAL_UNIT_ASSIGNED_CONTEXT((#459243,#459245,#459246))
REPRESENTATION_CONTEXT('','3D')
);
#459242=(
GEOMETRIC_REPRESENTATION_CONTEXT(3)
GLOBAL_UNCERTAINTY_ASSIGNED_CONTEXT((#459216))
GLOBAL_UNIT_ASSIGNED_CONTEXT((#459243,#459245,#459246))
REPRESENTATION_CONTEXT('','3D')
);
#459243=(
LENGTH_UNIT()
NAMED_UNIT(*)
SI_UNIT(.MILLI.,.METRE.)
);
#459245=(
NAMED_UNIT(*)
PLANE_ANGLE_UNIT()
SI_UNIT($,.RADIAN.)
);
#459246=(
NAMED_UNIT(*)
SI_UNIT($,.STERADIAN.)
SOLID_ANGLE_UNIT()
);
#459257=SHAPE_DEFINITION_REPRESENTATION(#459282,#459338);
#459282=PRODUCT_DEFINITION_SHAPE('',$,#459364);
#459338=SHAPE_REPRESENTATION('',(#98856),#459227);
#459353=PRODUCT_DEFINITION_CONTEXT('part definition',#459430,'design');
#459364=PRODUCT_DEFINITION('Needle Bearing','Needle Bearing',#459389,#459353);
#459389=PRODUCT_DEFINITION_FORMATION('',$,#459442);
#459430=APPLICATION_CONTEXT(
'Core Data for Automotive Mechanical Design Process');
#459431=PRODUCT_CONTEXT('part definition',#459430,'mechanical');
#459442=PRODUCT('Needle Bearing','Needle Bearing',$,(#459431));
#459520=COLOUR_RGB('Grey',0.48,0.52,0.57);
#459521=FILL_AREA_STYLE_COLOUR('',#459520);
#459522=FILL_AREA_STYLE('',(#459521));
#459523=SURFACE_STYLE_FILL_AREA(#459522);
#459524=SURFACE_SIDE_STYLE('',(#459523));
#459525=SURFACE_STYLE_USAGE(.BOTH.,#459524);
#459526=PRESENTATION_STYLE_ASSIGNMENT((#459525));
ENDSEC;
END-ISO-10303-21;
